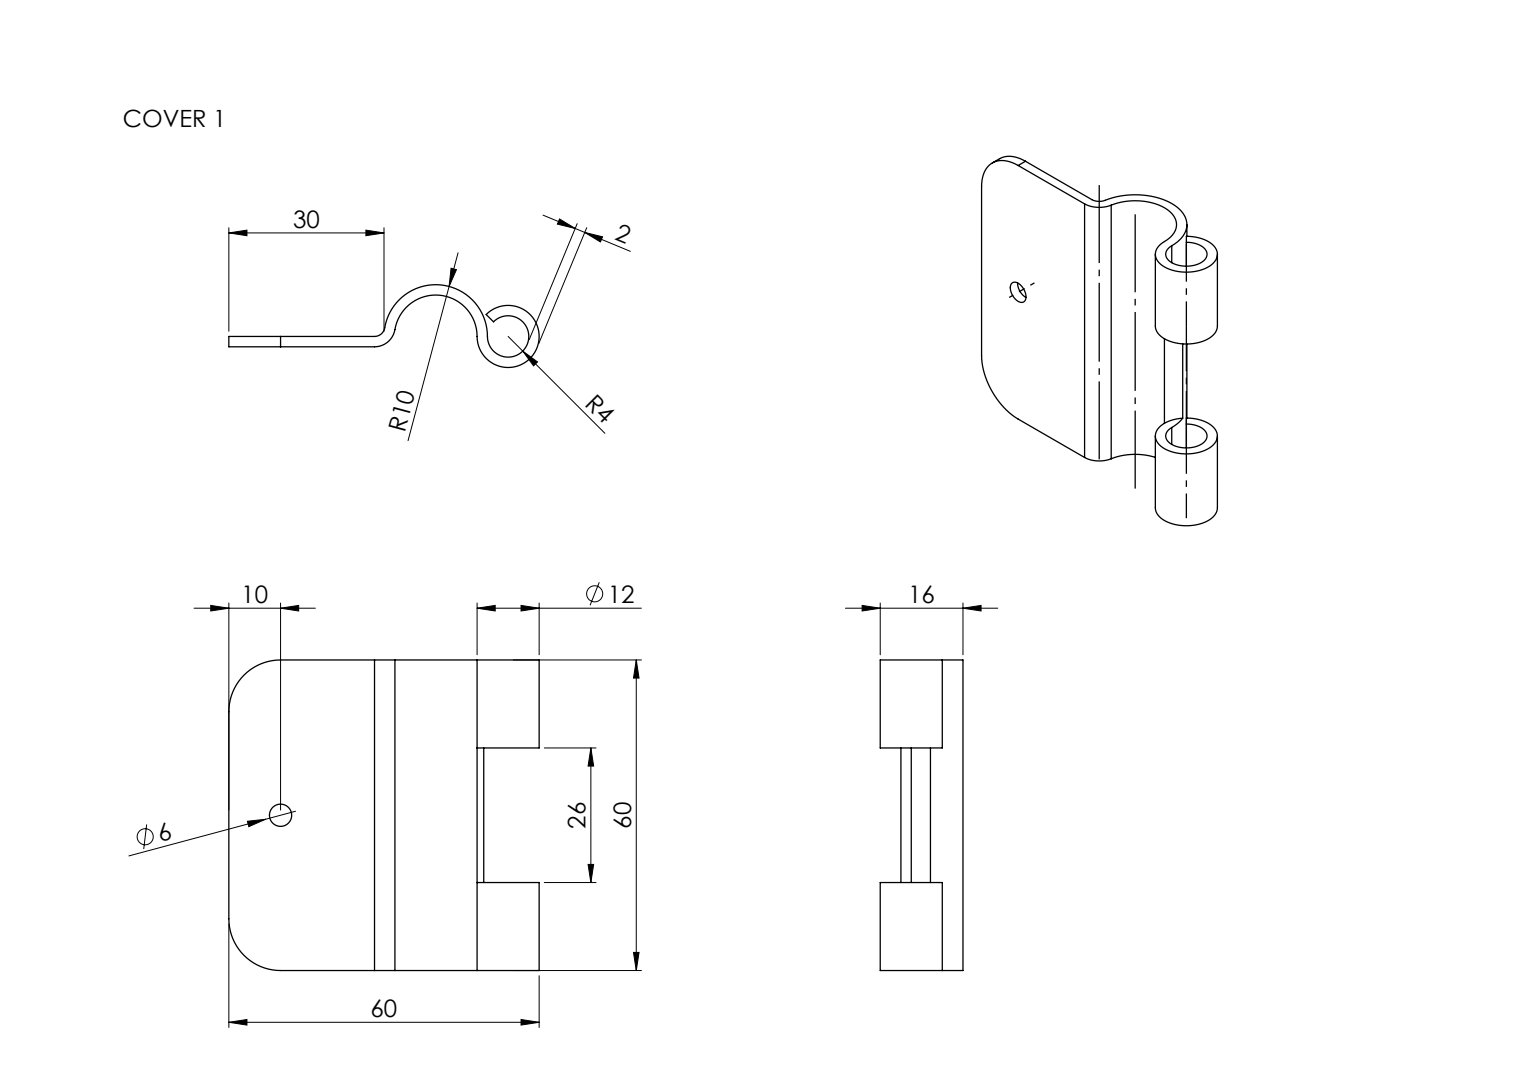
ISO-10303-21;
HEADER;
FILE_DESCRIPTION (('STEP AP214'),
    '1' );
FILE_NAME ('cover 1.step',
    '2026-10-03T20:08:58',
    ( '' ),
    ( '' ),
    'SwSTEP 2.0',
    'SolidWorks 2026',
    '' );
FILE_SCHEMA (( 'AUTOMOTIVE_DESIGN' ));
ENDSEC;

DATA;
#10=VECTOR ( 'NONE', #8821, 1000.000000000000000 ) ;
#24=LINE ( 'NONE', #10641, #9116 ) ;
#29=ORIENTED_EDGE ( 'NONE', *, *, #11225, .F. ) ;
#40=LINE ( 'NONE', #5122, #406 ) ;
#42=AXIS2_PLACEMENT_3D ( 'NONE', #12709, #3754, #3875 ) ;
#45=AXIS2_PLACEMENT_3D ( 'NONE', #142, #4066, #10040 ) ;
#48=DIRECTION ( 'NONE',  ( -0.000000000000000000, -1.000000000000000000, -0.000000000000000000 ) ) ;
#50=ORIENTED_EDGE ( 'NONE', *, *, #4393, .F. ) ;
#63=CARTESIAN_POINT ( 'NONE',  ( 14.00000000000000000, 12.99999999999999822, 0.000000000000000000 ) ) ;
#75=CARTESIAN_POINT ( 'NONE',  ( -11.83215956619923226, -30.00000000000000000, -4.336808689942017736E-16 ) ) ;
#77=DIRECTION ( 'NONE',  ( 0.000000000000000000, 0.000000000000000000, 1.000000000000000000 ) ) ;
#139=DIRECTION ( 'NONE',  ( 0.000000000000000000, 0.000000000000000000, -1.000000000000000000 ) ) ;
#142=CARTESIAN_POINT ( 'NONE',  ( 14.00000000000000000, 13.00000000000000000, 0.000000000000000000 ) ) ;
#148=CARTESIAN_POINT ( 'NONE',  ( 14.00000000000000000, -13.00000000000000000, 0.000000000000000000 ) ) ;
#158=ORIENTED_EDGE ( 'NONE', *, *, #7731, .T. ) ;
#171=AXIS2_PLACEMENT_3D ( 'NONE', #7633, #11626, #11439 ) ;
#181=ORIENTED_EDGE ( 'NONE', *, *, #9473, .F. ) ;
#187=AXIS2_PLACEMENT_3D ( 'NONE', #3419, #6498, #628 ) ;
#234=CIRCLE ( 'NONE', #8869, 6.000000000000000888 ) ;
#235=VERTEX_POINT ( 'NONE', #4529 ) ;
#237=EDGE_LOOP ( 'NONE', ( #1805, #3324, #10150, #7771, #10592, #866 ) ) ;
#273=CARTESIAN_POINT ( 'NONE',  ( 0.000000000000000000, 30.00000000000000000, 0.000000000000000000 ) ) ;
#288=AXIS2_PLACEMENT_3D ( 'NONE', #9402, #7554, #2747 ) ;
#294=DIRECTION ( 'NONE',  ( 0.000000000000000000, 0.000000000000000000, -1.000000000000000000 ) ) ;
#301=EDGE_LOOP ( 'NONE', ( #811, #8757, #4299, #181 ) ) ;
#303=VERTEX_POINT ( 'NONE', #7427 ) ;
#305=DIRECTION ( 'NONE',  ( -0.000000000000000000, -1.000000000000000000, -0.000000000000000000 ) ) ;
#333=EDGE_CURVE ( 'NONE', #5304, #561, #531, .T. ) ;
#344=DIRECTION ( 'NONE',  ( 0.000000000000000000, 0.000000000000000000, -1.000000000000000000 ) ) ;
#358=DIRECTION ( 'NONE',  ( 0.000000000000000000, 0.000000000000000000, 1.000000000000000000 ) ) ;
#377=ADVANCED_FACE ( 'NONE', ( #8824 ), #11672, .F. ) ;
#395=CARTESIAN_POINT ( 'NONE',  ( 14.00000000000000000, 12.99999999999999822, -4.000000000000000000 ) ) ;
#399=ORIENTED_EDGE ( 'NONE', *, *, #1607, .F. ) ;
#406=VECTOR ( 'NONE', #8142, 1000.000000000000000 ) ;
#412=VERTEX_POINT ( 'NONE', #4779 ) ;
#436=CARTESIAN_POINT ( 'NONE',  ( -11.83215956619923226, 30.00000000000000000, -4.336808689942017736E-16 ) ) ;
#444=VERTEX_POINT ( 'NONE', #9653 ) ;
#464=DIRECTION ( 'NONE',  ( 0.000000000000000000, 0.000000000000000000, -1.000000000000000000 ) ) ;
#469=DIRECTION ( 'NONE',  ( -1.000000000000000000, 0.000000000000000000, 1.301042606982605074E-16 ) ) ;
#475=ORIENTED_EDGE ( 'NONE', *, *, #9984, .T. ) ;
#476=CIRCLE ( 'NONE', #5414, 10.00000000000000178 ) ;
#531=LINE ( 'NONE', #9277, #10738 ) ;
#532=ADVANCED_FACE ( 'NONE', ( #11863 ), #11017, .F. ) ;
#535=DIRECTION ( 'NONE',  ( -0.000000000000000000, -1.000000000000000000, -0.000000000000000000 ) ) ;
#536=FACE_OUTER_BOUND ( 'NONE', #5367, .T. ) ;
#549=FACE_OUTER_BOUND ( 'NONE', #3644, .T. ) ;
#556=ORIENTED_EDGE ( 'NONE', *, *, #9689, .T. ) ;
#561=VERTEX_POINT ( 'NONE', #3052 ) ;
#617=ORIENTED_EDGE ( 'NONE', *, *, #7288, .T. ) ;
#628=DIRECTION ( 'NONE',  ( -1.000000000000000000, 0.000000000000000000, 1.159061634649218351E-16 ) ) ;
#638=DIRECTION ( 'NONE',  ( 0.000000000000000000, 1.000000000000000000, 0.000000000000000000 ) ) ;
#661=LINE ( 'NONE', #3823, #6580 ) ;
#672=DIRECTION ( 'NONE',  ( 0.000000000000000000, 0.000000000000000000, 1.000000000000000000 ) ) ;
#688=FACE_OUTER_BOUND ( 'NONE', #7012, .T. ) ;
#698=ORIENTED_EDGE ( 'NONE', *, *, #11571, .F. ) ;
#707=LINE ( 'NONE', #10430, #5346 ) ;
#711=VERTEX_POINT ( 'NONE', #7351 ) ;
#721=CARTESIAN_POINT ( 'NONE',  ( 14.00000000000000000, -12.99999999999999822, 0.000000000000000000 ) ) ;
#722=DIRECTION ( 'NONE',  ( -0.000000000000000000, 1.000000000000000000, 0.000000000000000000 ) ) ;
#727=CARTESIAN_POINT ( 'NONE',  ( 14.00000000000000000, -13.00000000000000000, 0.000000000000000000 ) ) ;
#729=VECTOR ( 'NONE', #11677, 1000.000000000000000 ) ;
#744=DIRECTION ( 'NONE',  ( 1.000000000000000000, 0.000000000000000000, 0.000000000000000000 ) ) ;
#751=AXIS2_PLACEMENT_3D ( 'NONE', #5443, #1637, #672 ) ;
#768=AXIS2_PLACEMENT_3D ( 'NONE', #5005, #48, #5840 ) ;
#771=DIRECTION ( 'NONE',  ( -0.000000000000000000, -1.000000000000000000, -0.000000000000000000 ) ) ;
#785=DIRECTION ( 'NONE',  ( 0.000000000000000000, 1.000000000000000000, 0.000000000000000000 ) ) ;
#803=VERTEX_POINT ( 'NONE', #3678 ) ;
#811=ORIENTED_EDGE ( 'NONE', *, *, #11377, .F. ) ;
#816=AXIS2_PLACEMENT_3D ( 'NONE', #12029, #3339, #7260 ) ;
#829=ORIENTED_EDGE ( 'NONE', *, *, #12238, .T. ) ;
#847=DIRECTION ( 'NONE',  ( 0.000000000000000000, 1.000000000000000000, 0.000000000000000000 ) ) ;
#866=ORIENTED_EDGE ( 'NONE', *, *, #11872, .F. ) ;
#898=AXIS2_PLACEMENT_3D ( 'NONE', #10933, #5615, #7679 ) ;
#924=DIRECTION ( 'NONE',  ( -0.000000000000000000, -1.000000000000000000, -0.000000000000000000 ) ) ;
#958=DIRECTION ( 'NONE',  ( 0.000000000000000000, 1.000000000000000000, 0.000000000000000000 ) ) ;
#971=LINE ( 'NONE', #75, #10203 ) ;
#974=LINE ( 'NONE', #5040, #7987 ) ;
#975=CIRCLE ( 'NONE', #6121, 2.000000000000000888 ) ;
#989=ORIENTED_EDGE ( 'NONE', *, *, #9398, .F. ) ;
#991=CARTESIAN_POINT ( 'NONE',  ( -30.00000000000000000, -19.99999999999999645, 0.000000000000000000 ) ) ;
#993=AXIS2_PLACEMENT_3D ( 'NONE', #148, #7994, #12663 ) ;
#998=DIRECTION ( 'NONE',  ( 0.000000000000000000, 0.000000000000000000, 1.000000000000000000 ) ) ;
#1000=ADVANCED_FACE ( 'NONE', ( #9168 ), #11180, .F. ) ;
#1016=ORIENTED_EDGE ( 'NONE', *, *, #5333, .F. ) ;
#1021=CIRCLE ( 'NONE', #8427, 4.000000000000000000 ) ;
#1034=CARTESIAN_POINT ( 'NONE',  ( -7.888106377466153063, -30.00000000000000000, -1.333333333333333703 ) ) ;
#1048=ADVANCED_FACE ( 'NONE', ( #9113 ), #5377, .T. ) ;
#1049=ADVANCED_FACE ( 'NONE', ( #8082 ), #8340, .T. ) ;
#1083=ADVANCED_FACE ( 'NONE', ( #549 ), #5630, .T. ) ;
#1111=ORIENTED_EDGE ( 'NONE', *, *, #9158, .T. ) ;
#1112=AXIS2_PLACEMENT_3D ( 'NONE', #1368, #344, #1244 ) ;
#1120=ORIENTED_EDGE ( 'NONE', *, *, #3514, .F. ) ;
#1127=ADVANCED_FACE ( 'NONE', ( #5693 ), #5574, .F. ) ;
#1155=ORIENTED_EDGE ( 'NONE', *, *, #3496, .F. ) ;
#1184=ORIENTED_EDGE ( 'NONE', *, *, #4506, .F. ) ;
#1193=FACE_BOUND ( 'NONE', #4343, .T. ) ;
#1200=ORIENTED_EDGE ( 'NONE', *, *, #2352, .F. ) ;
#1204=DIRECTION ( 'NONE',  ( -0.000000000000000000, -1.000000000000000000, -0.000000000000000000 ) ) ;
#1217=CARTESIAN_POINT ( 'NONE',  ( 9.999999999999998224, 30.00000000000000000, -6.123233995736765296E-16 ) ) ;
#1218=ORIENTED_EDGE ( 'NONE', *, *, #5875, .F. ) ;
#1242=CARTESIAN_POINT ( 'NONE',  ( -11.83215956619923226, -30.00000000000000000, -2.000000000000000888 ) ) ;
#1244=DIRECTION ( 'NONE',  ( -1.000000000000000000, 0.000000000000000000, 0.000000000000000000 ) ) ;
#1252=ORIENTED_EDGE ( 'NONE', *, *, #11293, .F. ) ;
#1255=PRESENTATION_STYLE_ASSIGNMENT (( #6281 ) ) ;
#1259=ADVANCED_FACE ( 'NONE', ( #4856 ), #6861, .F. ) ;
#1268=VECTOR ( 'NONE', #3945, 1000.000000000000000 ) ;
#1275=EDGE_CURVE ( 'NONE', #10532, #8740, #9012, .T. ) ;
#1283=DIRECTION ( 'NONE',  ( -0.000000000000000000, -1.000000000000000000, -0.000000000000000000 ) ) ;
#1287=ADVANCED_FACE ( 'NONE', ( #4920 ), #8781, .F. ) ;
#1288=CARTESIAN_POINT ( 'NONE',  ( 14.00000000000000000, -13.00000000000000000, 0.000000000000000000 ) ) ;
#1293=FACE_OUTER_BOUND ( 'NONE', #6936, .T. ) ;
#1307=APPLICATION_CONTEXT ( 'automotive_design' ) ;
#1309=CARTESIAN_POINT ( 'NONE',  ( -30.00000000000000000, 0.000000000000000000, 2.000000000000001776 ) ) ;
#1321=DIRECTION ( 'NONE',  ( 0.000000000000000000, 0.000000000000000000, -1.000000000000000000 ) ) ;
#1357=FACE_OUTER_BOUND ( 'NONE', #4922, .T. ) ;
#1368=CARTESIAN_POINT ( 'NONE',  ( -30.00000000000000000, 19.99999999999999645, 2.000000000000003109 ) ) ;
#1384=DIRECTION ( 'NONE',  ( -0.000000000000000000, -1.000000000000000000, -0.000000000000000000 ) ) ;
#1385=CARTESIAN_POINT ( 'NONE',  ( -27.85000000000000497, 2.632990618166801840E-16, 3.477184903947654954E-15 ) ) ;
#1404=CARTESIAN_POINT ( 'NONE',  ( -27.85000000000000853, 2.632990618166797895E-16, 2.185182530847200403E-15 ) ) ;
#1414=AXIS2_PLACEMENT_3D ( 'NONE', #436, #9498, #8356 ) ;
#1424=AXIS2_PLACEMENT_3D ( 'NONE', #12463, #7493, #4722 ) ;
#1426=AXIS2_PLACEMENT_3D ( 'NONE', #9293, #1384, #294 ) ;
#1444=CIRCLE ( 'NONE', #11915, 9.999999999999998224 ) ;
#1450=DIRECTION ( 'NONE',  ( -0.000000000000000000, -1.000000000000000000, -0.000000000000000000 ) ) ;
#1458=VERTEX_POINT ( 'NONE', #3664 ) ;
#1464=FACE_BOUND ( 'NONE', #5052, .T. ) ;
#1498=AXIS2_PLACEMENT_3D ( 'NONE', #11593, #2721, #9508 ) ;
#1523=ORIENTED_EDGE ( 'NONE', *, *, #4552, .F. ) ;
#1562=CYLINDRICAL_SURFACE ( 'NONE', #4873, 6.000000000000000000 ) ;
#1575=AXIS2_PLACEMENT_3D ( 'NONE', #1288, #10948, #10100 ) ;
#1580=CARTESIAN_POINT ( 'NONE',  ( 11.17157287525379772, 12.99999999999999822, -2.828427124746177856 ) ) ;
#1584=VERTEX_POINT ( 'NONE', #3083 ) ;
#1586=EDGE_LOOP ( 'NONE', ( #3626, #12343, #10983, #4232 ) ) ;
#1594=CARTESIAN_POINT ( 'NONE',  ( -40.00000000000000000, 19.99999999999999645, 2.000000000000003109 ) ) ;
#1607=EDGE_CURVE ( 'NONE', #3905, #2770, #8981, .T. ) ;
#1625=FACE_OUTER_BOUND ( 'NONE', #12477, .T. ) ;
#1637=DIRECTION ( 'NONE',  ( 0.000000000000000000, 1.000000000000000000, 0.000000000000000000 ) ) ;
#1641=EDGE_CURVE ( 'NONE', #3905, #1917, #6781, .T. ) ;
#1652=ORIENTED_EDGE ( 'NONE', *, *, #9989, .F. ) ;
#1655=SURFACE_SIDE_STYLE ('',( #4680 ) ) ;
#1661=VERTEX_POINT ( 'NONE', #4939 ) ;
#1670=CARTESIAN_POINT ( 'NONE',  ( 14.00000000000000000, -30.00000000000000000, 0.000000000000000000 ) ) ;
#1686=CIRCLE ( 'NONE', #45, 6.000000000000000888 ) ;
#1691=DIRECTION ( 'NONE',  ( -0.000000000000000000, -1.000000000000000000, -0.000000000000000000 ) ) ;
#1701=AXIS2_PLACEMENT_3D ( 'NONE', #5779, #5011, #9759 ) ;
#1790=AXIS2_PLACEMENT_3D ( 'NONE', #3328, #7245, #11163 ) ;
#1805=ORIENTED_EDGE ( 'NONE', *, *, #9881, .F. ) ;
#1817=DIRECTION ( 'NONE',  ( 0.000000000000000000, 0.000000000000000000, -1.000000000000000000 ) ) ;
#1820=EDGE_CURVE ( 'NONE', #6210, #11779, #1021, .T. ) ;
#1823=EDGE_LOOP ( 'NONE', ( #12079, #4616, #6876, #7646, #2549, #2027, #4556, #1218, #11515 ) ) ;
#1840=VECTOR ( 'NONE', #10679, 1000.000000000000000 ) ;
#1859=EDGE_CURVE ( 'NONE', #7604, #11454, #8226, .T. ) ;
#1885=AXIS2_PLACEMENT_3D ( 'NONE', #7237, #12196, #5357 ) ;
#1890=CARTESIAN_POINT ( 'NONE',  ( 14.00000000000000000, 30.00000000000000000, 0.000000000000000000 ) ) ;
#1895=CIRCLE ( 'NONE', #2324, 2.149999999999992362 ) ;
#1910=DIRECTION ( 'NONE',  ( 0.000000000000000000, -1.000000000000000000, 0.000000000000000000 ) ) ;
#1917=VERTEX_POINT ( 'NONE', #7123 ) ;
#1919=VECTOR ( 'NONE', #11565, 1000.000000000000000 ) ;
#1924=DIRECTION ( 'NONE',  ( -0.000000000000000000, -1.000000000000000000, -0.000000000000000000 ) ) ;
#1926=LINE ( 'NONE', #7854, #1840 ) ;
#1942=EDGE_CURVE ( 'NONE', #5074, #303, #40, .T. ) ;
#1953=CARTESIAN_POINT ( 'NONE',  ( -32.14999999999998437, 0.000000000000000000, 2.185182530847200403E-15 ) ) ;
#1960=AXIS2_PLACEMENT_3D ( 'NONE', #10965, #8263, #2155 ) ;
#1971=EDGE_LOOP ( 'NONE', ( #7157, #9270, #9490, #4872 ) ) ;
#1976=ORIENTED_EDGE ( 'NONE', *, *, #4473, .F. ) ;
#2027=ORIENTED_EDGE ( 'NONE', *, *, #11377, .T. ) ;
#2033=VECTOR ( 'NONE', #5157, 1000.000000000000000 ) ;
#2042=CIRCLE ( 'NONE', #6789, 6.000000000000000000 ) ;
#2057=CARTESIAN_POINT ( 'NONE',  ( 9.757359312880696578, 30.00000000000000000, -4.242640687119267007 ) ) ;
#2066=LINE ( 'NONE', #11735, #10 ) ;
#2073=LINE ( 'NONE', #5995, #4306 ) ;
#2106=PLANE ( 'NONE',  #5291 ) ;
#2117=CARTESIAN_POINT ( 'NONE',  ( -30.00000000000000000, 0.000000000000000000, 2.185182530847200403E-15 ) ) ;
#2155=DIRECTION ( 'NONE',  ( 0.000000000000000000, 0.000000000000000000, -1.000000000000000000 ) ) ;
#2157=LINE ( 'NONE', #3013, #9658 ) ;
#2158=ORIENTED_EDGE ( 'NONE', *, *, #3957, .T. ) ;
#2174=DIRECTION ( 'NONE',  ( -0.000000000000000000, -0.000000000000000000, -1.000000000000000000 ) ) ;
#2183=EDGE_LOOP ( 'NONE', ( #11415, #8143, #11917, #10065 ) ) ;
#2184=EDGE_CURVE ( 'NONE', #9120, #8530, #2066, .T. ) ;
#2214=ORIENTED_EDGE ( 'NONE', *, *, #6084, .F. ) ;
#2240=ORIENTED_EDGE ( 'NONE', *, *, #1641, .F. ) ;
#2258=DIRECTION ( 'NONE',  ( 1.000000000000000000, 0.000000000000000000, 0.000000000000000000 ) ) ;
#2265=PLANE ( 'NONE',  #4114 ) ;
#2284=COLOUR_RGB ( '', 0.72549020, 0.75294118, 0.79215686) ;
#2299=ORIENTED_EDGE ( 'NONE', *, *, #5405, .F. ) ;
#2310=ORIENTED_EDGE ( 'NONE', *, *, #5875, .T. ) ;
#2324=AXIS2_PLACEMENT_3D ( 'NONE', #9320, #4378, #10287 ) ;
#2332=AXIS2_PLACEMENT_3D ( 'NONE', #1670, #638, #4577 ) ;
#2333=CARTESIAN_POINT ( 'NONE',  ( 14.00000000000000000, 30.00000000000000000, 0.000000000000000000 ) ) ;
#2336=FACE_OUTER_BOUND ( 'NONE', #3673, .T. ) ;
#2352=EDGE_CURVE ( 'NONE', #1661, #235, #12058, .T. ) ;
#2381=ORIENTED_EDGE ( 'NONE', *, *, #2850, .T. ) ;
#2382=DIRECTION ( 'NONE',  ( 0.000000000000000000, 0.000000000000000000, 1.000000000000000000 ) ) ;
#2387=ADVANCED_FACE ( 'NONE', ( #4252 ), #2265, .F. ) ;
#2391=ORIENTED_EDGE ( 'NONE', *, *, #2184, .T. ) ;
#2392=AXIS2_PLACEMENT_3D ( 'NONE', #6722, #12712, #5872 ) ;
#2416=PRODUCT_DEFINITION_FORMATION_WITH_SPECIFIED_SOURCE ( 'ANY', '', #6601, .NOT_KNOWN. ) ;
#2417=AXIS2_PLACEMENT_3D ( 'NONE', #721, #847, #10566 ) ;
#2426=VECTOR ( 'NONE', #3154, 1000.000000000000000 ) ;
#2438=ORIENTED_EDGE ( 'NONE', *, *, #10969, .T. ) ;
#2444=FACE_OUTER_BOUND ( 'NONE', #7944, .T. ) ;
#2461=AXIS2_PLACEMENT_3D ( 'NONE', #8419, #9369, #7579 ) ;
#2465=FACE_OUTER_BOUND ( 'NONE', #10736, .T. ) ;
#2476=CARTESIAN_POINT ( 'NONE',  ( 14.00000000000000000, 30.00000000000000000, 6.000000000000000000 ) ) ;
#2493=CARTESIAN_POINT ( 'NONE',  ( -30.00000000000000000, -19.99999999999999645, 2.000000000000001776 ) ) ;
#2495=DIRECTION ( 'NONE',  ( 0.000000000000000000, 0.000000000000000000, -1.000000000000000000 ) ) ;
#2509=DIRECTION ( 'NONE',  ( 0.000000000000000000, 0.000000000000000000, -1.000000000000000000 ) ) ;
#2537=CIRCLE ( 'NONE', #2332, 6.000000000000000000 ) ;
#2549=ORIENTED_EDGE ( 'NONE', *, *, #5470, .T. ) ;
#2572=ORIENTED_EDGE ( 'NONE', *, *, #7361, .F. ) ;
#2574=CARTESIAN_POINT ( 'NONE',  ( 0.000000000000000000, -30.00000000000000000, 0.000000000000000000 ) ) ;
#2600=ORIENTED_EDGE ( 'NONE', *, *, #7623, .F. ) ;
#2611=STYLED_ITEM ( 'NONE', ( #1255 ), #5784 ) ;
#2664=DIRECTION ( 'NONE',  ( -0.000000000000000000, -1.000000000000000000, -0.000000000000000000 ) ) ;
#2676=CARTESIAN_POINT ( 'NONE',  ( 11.17157287525379772, 30.00000000000000000, -2.828427124746177856 ) ) ;
#2704=ORIENTED_EDGE ( 'NONE', *, *, #3659, .F. ) ;
#2716=CARTESIAN_POINT ( 'NONE',  ( 14.00000000000000000, -30.00000000000000000, 6.000000000000000000 ) ) ;
#2721=DIRECTION ( 'NONE',  ( 0.000000000000000000, 1.000000000000000000, 0.000000000000000000 ) ) ;
#2745=DIRECTION ( 'NONE',  ( 1.000000000000000000, 0.000000000000000000, 0.000000000000000000 ) ) ;
#2747=DIRECTION ( 'NONE',  ( -1.000000000000000000, 0.000000000000000000, 0.000000000000000000 ) ) ;
#2751=EDGE_CURVE ( 'NONE', #11755, #9393, #12335, .T. ) ;
#2770=VERTEX_POINT ( 'NONE', #4043 ) ;
#2782=VERTEX_POINT ( 'NONE', #5267 ) ;
#2805=DIRECTION ( 'NONE',  ( 1.000000000000000000, 0.000000000000000000, -1.159061634649218351E-16 ) ) ;
#2809=DIRECTION ( 'NONE',  ( -0.7071067811865504593, 0.000000000000000000, -0.7071067811865445751 ) ) ;
#2810=ADVANCED_FACE ( 'NONE', ( #8032 ), #11066, .T. ) ;
#2818=VERTEX_POINT ( 'NONE', #9125 ) ;
#2843=ADVANCED_FACE ( 'NONE', ( #1464, #2444 ), #5588, .T. ) ;
#2850=EDGE_CURVE ( 'NONE', #5717, #8530, #1444, .T. ) ;
#2878=ADVANCED_FACE ( 'NONE', ( #688 ), #11522, .F. ) ;
#2901=CARTESIAN_POINT ( 'NONE',  ( 14.00000000000000000, -13.00000000000000000, 0.000000000000000000 ) ) ;
#2904=PRODUCT_DEFINITION ( 'UNKNOWN', '', #2416, #10936 ) ;
#2917=VECTOR ( 'NONE', #9738, 1000.000000000000000 ) ;
#2921=EDGE_CURVE ( 'NONE', #561, #2818, #5738, .T. ) ;
#2937=CARTESIAN_POINT ( 'NONE',  ( 14.00000000000000000, 30.00000000000000000, 4.000000000000000000 ) ) ;
#2941=VERTEX_POINT ( 'NONE', #5525 ) ;
#2943=DIRECTION ( 'NONE',  ( -0.000000000000000000, -1.000000000000000000, -0.000000000000000000 ) ) ;
#2953=ORIENTED_EDGE ( 'NONE', *, *, #9013, .F. ) ;
#2970=ORIENTED_EDGE ( 'NONE', *, *, #1859, .T. ) ;
#2976=ORIENTED_EDGE ( 'NONE', *, *, #4473, .T. ) ;
#2980=DIRECTION ( 'NONE',  ( 0.000000000000000000, 0.000000000000000000, 1.000000000000000000 ) ) ;
#3013=CARTESIAN_POINT ( 'NONE',  ( -7.888106377466153063, 30.00000000000000000, -1.333333333333333703 ) ) ;
#3023=VERTEX_POINT ( 'NONE', #12618 ) ;
#3032=ORIENTED_EDGE ( 'NONE', *, *, #5231, .T. ) ;
#3042=AXIS2_PLACEMENT_3D ( 'NONE', #3819, #3939, #6595 ) ;
#3052=CARTESIAN_POINT ( 'NONE',  ( -29.99999999999999289, -30.00000000000000000, 1.672083814130525448E-15 ) ) ;
#3054=EDGE_CURVE ( 'NONE', #803, #11695, #6235, .T. ) ;
#3070=EDGE_CURVE ( 'NONE', #3108, #11779, #5837, .T. ) ;
#3071=CARTESIAN_POINT ( 'NONE',  ( 0.000000000000000000, -30.00000000000000000, -9.999999999999998224 ) ) ;
#3082=VERTEX_POINT ( 'NONE', #10788 ) ;
#3083=CARTESIAN_POINT ( 'NONE',  ( 9.999999999999998224, -30.00000000000000000, -6.123233995736765296E-16 ) ) ;
#3085=ORIENTED_EDGE ( 'NONE', *, *, #6575, .T. ) ;
#3092=ORIENTED_EDGE ( 'NONE', *, *, #4506, .T. ) ;
#3103=CIRCLE ( 'NONE', #11936, 6.000000000000000000 ) ;
#3108=VERTEX_POINT ( 'NONE', #7649 ) ;
#3125=VECTOR ( 'NONE', #11827, 1000.000000000000000 ) ;
#3138=VECTOR ( 'NONE', #2664, 1000.000000000000000 ) ;
#3154=DIRECTION ( 'NONE',  ( -0.000000000000000000, -1.000000000000000000, -0.000000000000000000 ) ) ;
#3174=DIRECTION ( 'NONE',  ( 0.000000000000000000, 1.000000000000000000, 0.000000000000000000 ) ) ;
#3177=CIRCLE ( 'NONE', #5625, 7.999999999999998224 ) ;
#3197=DIRECTION ( 'NONE',  ( 0.000000000000000000, 1.000000000000000000, 0.000000000000000000 ) ) ;
#3245=DIRECTION ( 'NONE',  ( -1.000000000000000000, 0.000000000000000000, 0.000000000000000000 ) ) ;
#3247=CIRCLE ( 'NONE', #3042, 6.000000000000000000 ) ;
#3255=VECTOR ( 'NONE', #5993, 1000.000000000000000 ) ;
#3262=DIRECTION ( 'NONE',  ( 1.000000000000000000, 0.000000000000000000, 0.000000000000000000 ) ) ;
#3265=CIRCLE ( 'NONE', #10433, 9.999999999999998224 ) ;
#3284=ORIENTED_EDGE ( 'NONE', *, *, #12203, .T. ) ;
#3296=CARTESIAN_POINT ( 'NONE',  ( 11.17157287525379772, -12.99999999999999822, -2.828427124746177856 ) ) ;
#3302=CARTESIAN_POINT ( 'NONE',  ( -40.00000000000000000, 19.99999999999999645, 2.831145448779744488E-15 ) ) ;
#3318=DIRECTION ( 'NONE',  ( 0.000000000000000000, 1.000000000000000000, 0.000000000000000000 ) ) ;
#3320=CARTESIAN_POINT ( 'NONE',  ( -11.83215956619923226, 30.00000000000000000, 2.000000000000000000 ) ) ;
#3324=ORIENTED_EDGE ( 'NONE', *, *, #7361, .T. ) ;
#3328=CARTESIAN_POINT ( 'NONE',  ( 0.000000000000000000, 30.00000000000000000, 0.000000000000000000 ) ) ;
#3339=DIRECTION ( 'NONE',  ( -0.000000000000000000, -1.000000000000000000, -0.000000000000000000 ) ) ;
#3340=DIRECTION ( 'NONE',  ( -1.159061634649218351E-16, 0.000000000000000000, -1.000000000000000000 ) ) ;
#3376=CARTESIAN_POINT ( 'NONE',  ( 0.000000000000000000, 30.00000000000000000, -9.999999999999998224 ) ) ;
#3377=ORIENTED_EDGE ( 'NONE', *, *, #11293, .T. ) ;
#3381=EDGE_CURVE ( 'NONE', #235, #5304, #476, .T. ) ;
#3419=CARTESIAN_POINT ( 'NONE',  ( -30.00000000000000000, -19.99999999999999645, 1.672083814130526039E-15 ) ) ;
#3435=LINE ( 'NONE', #7353, #4862 ) ;
#3440=DIRECTION ( 'NONE',  ( -0.000000000000000000, -1.000000000000000000, -0.000000000000000000 ) ) ;
#3449=FACE_OUTER_BOUND ( 'NONE', #301, .T. ) ;
#3464=ADVANCED_FACE ( 'NONE', ( #3829 ), #6609, .F. ) ;
#3488=DIRECTION ( 'NONE',  ( -1.000000000000000000, 0.000000000000000000, 0.000000000000000000 ) ) ;
#3496=EDGE_CURVE ( 'NONE', #12099, #5977, #24, .T. ) ;
#3504=ORIENTED_EDGE ( 'NONE', *, *, #8796, .F. ) ;
#3508=CARTESIAN_POINT ( 'NONE',  ( 14.00000000000000000, 30.00000000000000000, 0.000000000000000000 ) ) ;
#3514=EDGE_CURVE ( 'NONE', #5304, #8798, #7631, .T. ) ;
#3530=EDGE_LOOP ( 'NONE', ( #3597, #9990, #8842, #11421 ) ) ;
#3537=ORIENTED_EDGE ( 'NONE', *, *, #4198, .F. ) ;
#3567=ORIENTED_EDGE ( 'NONE', *, *, #7143, .T. ) ;
#3574=VECTOR ( 'NONE', #12296, 1000.000000000000000 ) ;
#3582=ORIENTED_EDGE ( 'NONE', *, *, #10353, .T. ) ;
#3593=ORIENTED_EDGE ( 'NONE', *, *, #7143, .F. ) ;
#3597=ORIENTED_EDGE ( 'NONE', *, *, #12203, .F. ) ;
#3626=ORIENTED_EDGE ( 'NONE', *, *, #5180, .F. ) ;
#3638=UNCERTAINTY_MEASURE_WITH_UNIT (LENGTH_MEASURE( 1.000000000000000082E-05 ), #10533, 'distance_accuracy_value', 'NONE');
#3644=EDGE_LOOP ( 'NONE', ( #10651, #8593, #5758, #8809 ) ) ;
#3659=EDGE_CURVE ( 'NONE', #1458, #2782, #3177, .T. ) ;
#3664=CARTESIAN_POINT ( 'NONE',  ( -7.888106377466153063, 30.00000000000000000, -1.333333333333333703 ) ) ;
#3673=EDGE_LOOP ( 'NONE', ( #4612, #9882, #9043, #10462 ) ) ;
#3678=CARTESIAN_POINT ( 'NONE',  ( 14.00000000000000000, 12.99999999999999822, 4.000000000000000000 ) ) ;
#3702=DIRECTION ( 'NONE',  ( 0.000000000000000000, 1.000000000000000000, 0.000000000000000000 ) ) ;
#3711=VECTOR ( 'NONE', #6854, 1000.000000000000000 ) ;
#3754=DIRECTION ( 'NONE',  ( -0.000000000000000000, -1.000000000000000000, -0.000000000000000000 ) ) ;
#3758=CARTESIAN_POINT ( 'NONE',  ( 0.000000000000000000, -30.00000000000000000, 0.000000000000000000 ) ) ;
#3776=ORIENTED_EDGE ( 'NONE', *, *, #5299, .F. ) ;
#3789=CARTESIAN_POINT ( 'NONE',  ( 0.000000000000000000, 30.00000000000000000, 0.000000000000000000 ) ) ;
#3819=CARTESIAN_POINT ( 'NONE',  ( 14.00000000000000000, 30.00000000000000000, 0.000000000000000000 ) ) ;
#3823=CARTESIAN_POINT ( 'NONE',  ( 11.17157287525379772, 30.00000000000000000, -2.828427124746177856 ) ) ;
#3829=FACE_OUTER_BOUND ( 'NONE', #11908, .T. ) ;
#3839=ORIENTED_EDGE ( 'NONE', *, *, #7448, .F. ) ;
#3846=ORIENTED_EDGE ( 'NONE', *, *, #1942, .F. ) ;
#3861=VERTEX_POINT ( 'NONE', #8578 ) ;
#3875=DIRECTION ( 'NONE',  ( 0.000000000000000000, 0.000000000000000000, -1.000000000000000000 ) ) ;
#3879=DIRECTION ( 'NONE',  ( 1.000000000000000000, 0.000000000000000000, 0.000000000000000000 ) ) ;
#3897=AXIS2_PLACEMENT_3D ( 'NONE', #11809, #5102, #139 ) ;
#3905=VERTEX_POINT ( 'NONE', #12585 ) ;
#3909=CIRCLE ( 'NONE', #6799, 4.000000000000000000 ) ;
#3923=VERTEX_POINT ( 'NONE', #4045 ) ;
#3939=DIRECTION ( 'NONE',  ( 0.000000000000000000, 1.000000000000000000, 0.000000000000000000 ) ) ;
#3945=DIRECTION ( 'NONE',  ( -0.000000000000000000, -0.000000000000000000, 1.000000000000000000 ) ) ;
#3957=EDGE_CURVE ( 'NONE', #11695, #711, #8923, .T. ) ;
#3968=CARTESIAN_POINT ( 'NONE',  ( 0.000000000000000000, -30.00000000000000000, 0.000000000000000000 ) ) ;
#3987=CYLINDRICAL_SURFACE ( 'NONE', #10792, 4.000000000000000000 ) ;
#4020=VERTEX_POINT ( 'NONE', #3296 ) ;
#4021=AXIS2_PLACEMENT_3D ( 'NONE', #1242, #4271, #12142 ) ;
#4043=CARTESIAN_POINT ( 'NONE',  ( 8.000000000000000000, -30.00000000000000000, -7.347880794884119736E-16 ) ) ;
#4045=CARTESIAN_POINT ( 'NONE',  ( 9.999999999999998224, 30.00000000000000000, -6.123233995736765296E-16 ) ) ;
#4066=DIRECTION ( 'NONE',  ( 0.000000000000000000, 1.000000000000000000, 0.000000000000000000 ) ) ;
#4094=LINE ( 'NONE', #12030, #2426 ) ;
#4114=AXIS2_PLACEMENT_3D ( 'NONE', #10944, #7286, #11212 ) ;
#4143=EDGE_LOOP ( 'NONE', ( #1120, #9739, #12659, #12338, #2381, #6160, #6958, #10639, #3567, #12272, #8998, #8819, #9422, #4803, #7145, #7439 ) ) ;
#4164=DIRECTION ( 'NONE',  ( 0.000000000000000000, 1.000000000000000000, 0.000000000000000000 ) ) ;
#4185=CARTESIAN_POINT ( 'NONE',  ( 14.00000000000000000, 13.00000000000000000, 0.000000000000000000 ) ) ;
#4198=EDGE_CURVE ( 'NONE', #1661, #9551, #10408, .T. ) ;
#4208=ORIENTED_EDGE ( 'NONE', *, *, #3054, .F. ) ;
#4216=AXIS2_PLACEMENT_3D ( 'NONE', #63, #958, #2980 ) ;
#4228=CIRCLE ( 'NONE', #4021, 4.000000000000000000 ) ;
#4232=ORIENTED_EDGE ( 'NONE', *, *, #8987, .F. ) ;
#4235=CARTESIAN_POINT ( 'NONE',  ( 11.17157287525379772, -30.00000000000000000, -2.828427124746177856 ) ) ;
#4237=EDGE_LOOP ( 'NONE', ( #3504, #10227, #11106, #1111, #4887, #11159, #5172, #4346, #12022, #1652, #5776, #7252, #6142, #50, #7426, #10177 ) ) ;
#4246=CARTESIAN_POINT ( 'NONE',  ( 14.00000000000000000, -30.00000000000000000, 0.000000000000000000 ) ) ;
#4249=DIRECTION ( 'NONE',  ( 0.000000000000000000, 1.000000000000000000, 0.000000000000000000 ) ) ;
#4252=FACE_OUTER_BOUND ( 'NONE', #4143, .T. ) ;
#4271=DIRECTION ( 'NONE',  ( 0.000000000000000000, 1.000000000000000000, 0.000000000000000000 ) ) ;
#4276=VERTEX_POINT ( 'NONE', #10540 ) ;
#4295=LINE ( 'NONE', #9306, #5212 ) ;
#4299=ORIENTED_EDGE ( 'NONE', *, *, #12320, .T. ) ;
#4306=VECTOR ( 'NONE', #7806, 1000.000000000000000 ) ;
#4328=EDGE_CURVE ( 'NONE', #11755, #7484, #11060, .T. ) ;
#4343=EDGE_LOOP ( 'NONE', ( #3377, #3284 ) ) ;
#4346=ORIENTED_EDGE ( 'NONE', *, *, #5180, .T. ) ;
#4359=ORIENTED_EDGE ( 'NONE', *, *, #9569, .T. ) ;
#4364=CARTESIAN_POINT ( 'NONE',  ( -9.860132971832690885, -30.00000000000000000, -1.666666666666667629 ) ) ;
#4366=APPLICATION_CONTEXT ( 'automotive_design' ) ;
#4370=DIRECTION ( 'NONE',  ( 0.000000000000000000, 1.000000000000000000, 0.000000000000000000 ) ) ;
#4377=ORIENTED_EDGE ( 'NONE', *, *, #9013, .T. ) ;
#4378=DIRECTION ( 'NONE',  ( -1.159061634649218351E-16, 0.000000000000000000, -1.000000000000000000 ) ) ;
#4393=EDGE_CURVE ( 'NONE', #9120, #3923, #3265, .T. ) ;
#4400=DIRECTION ( 'NONE',  ( 0.000000000000000000, 0.000000000000000000, -1.000000000000000000 ) ) ;
#4426=LINE ( 'NONE', #8351, #3574 ) ;
#4463=CARTESIAN_POINT ( 'NONE',  ( 14.00000000000000000, -30.00000000000000000, 4.000000000000000000 ) ) ;
#4473=EDGE_CURVE ( 'NONE', #9408, #412, #12100, .T. ) ;
#4478=ORIENTED_EDGE ( 'NONE', *, *, #7288, .F. ) ;
#4483=EDGE_CURVE ( 'NONE', #9770, #5717, #975, .T. ) ;
#4488=CARTESIAN_POINT ( 'NONE',  ( -40.00000000000000000, 30.00000000000000000, 2.831145448779744488E-15 ) ) ;
#4489=VERTEX_POINT ( 'NONE', #8022 ) ;
#4506=EDGE_CURVE ( 'NONE', #2782, #11454, #4094, .T. ) ;
#4513=AXIS2_PLACEMENT_3D ( 'NONE', #10931, #1204, #11980 ) ;
#4526=ADVANCED_FACE ( 'NONE', ( #1193, #6154 ), #2106, .F. ) ;
#4529=CARTESIAN_POINT ( 'NONE',  ( -40.00000000000000000, -19.99999999999999645, 2.000000000000003109 ) ) ;
#4531=CARTESIAN_POINT ( 'NONE',  ( 14.00000000000000000, 30.00000000000000000, 4.000000000000000000 ) ) ;
#4549=DIRECTION ( 'NONE',  ( -0.000000000000000000, -1.000000000000000000, -0.000000000000000000 ) ) ;
#4552=EDGE_CURVE ( 'NONE', #4276, #8365, #10987, .T. ) ;
#4556=ORIENTED_EDGE ( 'NONE', *, *, #9984, .F. ) ;
#4574=ORIENTED_EDGE ( 'NONE', *, *, #11571, .T. ) ;
#4576=EDGE_LOOP ( 'NONE', ( #1184, #2704, #11370, #2970 ) ) ;
#4577=DIRECTION ( 'NONE',  ( 1.000000000000000000, 0.000000000000000000, 0.000000000000000000 ) ) ;
#4612=ORIENTED_EDGE ( 'NONE', *, *, #7383, .T. ) ;
#4616=ORIENTED_EDGE ( 'NONE', *, *, #12238, .F. ) ;
#4629=CIRCLE ( 'NONE', #10779, 4.000000000000000000 ) ;
#4641=AXIS2_PLACEMENT_3D ( 'NONE', #11442, #12353, #4741 ) ;
#4644=PRODUCT_DEFINITION_SHAPE ( 'NONE', 'NONE',  #2904 ) ;
#4680=SURFACE_STYLE_FILL_AREA ( #10335 ) ;
#4714=AXIS2_PLACEMENT_3D ( 'NONE', #7018, #5329, #2382 ) ;
#4722=DIRECTION ( 'NONE',  ( 0.000000000000000000, 0.000000000000000000, 1.000000000000000000 ) ) ;
#4741=DIRECTION ( 'NONE',  ( 0.000000000000000000, 0.000000000000000000, 1.000000000000000000 ) ) ;
#4747=MECHANICAL_DESIGN_GEOMETRIC_PRESENTATION_REPRESENTATION('',(#11741),#5160);
#4751=SURFACE_STYLE_USAGE ( .BOTH. , #1655 ) ;
#4765=CIRCLE ( 'NONE', #5370, 2.149999999999992362 ) ;
#4779=CARTESIAN_POINT ( 'NONE',  ( 9.757359312880696578, 13.00000000000000000, -4.242640687119267895 ) ) ;
#4786=CIRCLE ( 'NONE', #6022, 2.149999999999985256 ) ;
#4803=ORIENTED_EDGE ( 'NONE', *, *, #7731, .F. ) ;
#4828=AXIS2_PLACEMENT_3D ( 'NONE', #7278, #4370, #11200 ) ;
#4835=VERTEX_POINT ( 'NONE', #1953 ) ;
#4844=AXIS2_PLACEMENT_3D ( 'NONE', #9985, #6139, #469 ) ;
#4856=FACE_OUTER_BOUND ( 'NONE', #11883, .T. ) ;
#4862=VECTOR ( 'NONE', #7231, 1000.000000000000000 ) ;
#4863=LINE ( 'NONE', #12730, #7831 ) ;
#4872=ORIENTED_EDGE ( 'NONE', *, *, #3957, .F. ) ;
#4873=AXIS2_PLACEMENT_3D ( 'NONE', #3508, #535, #4400 ) ;
#4887=ORIENTED_EDGE ( 'NONE', *, *, #3659, .T. ) ;
#4915=CARTESIAN_POINT ( 'NONE',  ( 14.00000000000000000, 30.00000000000000000, 0.000000000000000000 ) ) ;
#4920=FACE_OUTER_BOUND ( 'NONE', #10327, .T. ) ;
#4922=EDGE_LOOP ( 'NONE', ( #6338, #11445, #2976, #10317 ) ) ;
#4931=LINE ( 'NONE', #8851, #3125 ) ;
#4939=CARTESIAN_POINT ( 'NONE',  ( -40.00000000000000000, 19.99999999999999645, 2.000000000000003109 ) ) ;
#4960=ORIENTED_EDGE ( 'NONE', *, *, #10619, .T. ) ;
#4987=CARTESIAN_POINT ( 'NONE',  ( 8.000000000000000000, 30.00000000000000000, -7.347880794884119736E-16 ) ) ;
#5005=CARTESIAN_POINT ( 'NONE',  ( 0.000000000000000000, 12.99999999999999822, 0.000000000000000000 ) ) ;
#5011=DIRECTION ( 'NONE',  ( -0.000000000000000000, -0.000000000000000000, -1.000000000000000000 ) ) ;
#5020=EDGE_CURVE ( 'NONE', #2782, #6170, #11463, .T. ) ;
#5040=CARTESIAN_POINT ( 'NONE',  ( -11.83215956619923226, 30.00000000000000000, -4.336808689942017736E-16 ) ) ;
#5052=EDGE_LOOP ( 'NONE', ( #12492, #6427 ) ) ;
#5053=ADVANCED_FACE ( 'NONE', ( #3449 ), #1562, .T. ) ;
#5056=DIRECTION ( 'NONE',  ( -0.000000000000000000, -1.000000000000000000, -0.000000000000000000 ) ) ;
#5074=VERTEX_POINT ( 'NONE', #2476 ) ;
#5102=DIRECTION ( 'NONE',  ( 0.000000000000000000, -1.000000000000000000, 0.000000000000000000 ) ) ;
#5106=ORIENTED_EDGE ( 'NONE', *, *, #7627, .T. ) ;
#5109=AXIS2_PLACEMENT_3D ( 'NONE', #10187, #1450, #2495 ) ;
#5122=CARTESIAN_POINT ( 'NONE',  ( 14.00000000000000000, 30.00000000000000000, 6.000000000000000000 ) ) ;
#5130=( NAMED_UNIT ( * ) SI_UNIT ( $, .STERADIAN. ) SOLID_ANGLE_UNIT ( ) );
#5157=DIRECTION ( 'NONE',  ( -0.000000000000000000, -1.000000000000000000, -0.000000000000000000 ) ) ;
#5158=ORIENTED_EDGE ( 'NONE', *, *, #10844, .T. ) ;
#5159=CARTESIAN_POINT ( 'NONE',  ( -30.00000000000000000, 0.000000000000000000, 3.477184903947654954E-15 ) ) ;
#5160=( GEOMETRIC_REPRESENTATION_CONTEXT ( 3 ) GLOBAL_UNCERTAINTY_ASSIGNED_CONTEXT ( ( #11617 ) ) GLOBAL_UNIT_ASSIGNED_CONTEXT ( ( #12424, #11452, #12364 ) ) REPRESENTATION_CONTEXT ( 'NONE', 'WORKASPACE' ) );
#5172=ORIENTED_EDGE ( 'NONE', *, *, #6084, .T. ) ;
#5174=DIRECTION ( 'NONE',  ( 1.000000000000000000, 0.000000000000000000, 0.000000000000000000 ) ) ;
#5180=EDGE_CURVE ( 'NONE', #5074, #6567, #3247, .T. ) ;
#5188=ORIENTED_EDGE ( 'NONE', *, *, #2751, .T. ) ;
#5199=ORIENTED_EDGE ( 'NONE', *, *, #11225, .T. ) ;
#5212=VECTOR ( 'NONE', #305, 1000.000000000000000 ) ;
#5231=EDGE_CURVE ( 'NONE', #4489, #12605, #11669, .T. ) ;
#5255=DIRECTION ( 'NONE',  ( -0.000000000000000000, -1.000000000000000000, -0.000000000000000000 ) ) ;
#5267=CARTESIAN_POINT ( 'NONE',  ( 0.000000000000000000, 30.00000000000000000, -7.999999999999998224 ) ) ;
#5283=EDGE_CURVE ( 'NONE', #8740, #711, #6849, .T. ) ;
#5291=AXIS2_PLACEMENT_3D ( 'NONE', #7957, #3340, #10189 ) ;
#5299=EDGE_CURVE ( 'NONE', #9551, #12099, #10625, .T. ) ;
#5304=VERTEX_POINT ( 'NONE', #7922 ) ;
#5312=( LENGTH_UNIT ( ) NAMED_UNIT ( * ) SI_UNIT ( .MILLI., .METRE. ) );
#5329=DIRECTION ( 'NONE',  ( 0.000000000000000000, 1.000000000000000000, 0.000000000000000000 ) ) ;
#5333=EDGE_CURVE ( 'NONE', #2941, #3905, #12075, .T. ) ;
#5343=DIRECTION ( 'NONE',  ( -0.000000000000000000, -1.000000000000000000, -0.000000000000000000 ) ) ;
#5346=VECTOR ( 'NONE', #771, 1000.000000000000000 ) ;
#5357=DIRECTION ( 'NONE',  ( 0.000000000000000000, 0.000000000000000000, -1.000000000000000000 ) ) ;
#5367=EDGE_LOOP ( 'NONE', ( #11973, #4960, #3085, #989 ) ) ;
#5370=AXIS2_PLACEMENT_3D ( 'NONE', #1309, #5434, #9286 ) ;
#5377=CYLINDRICAL_SURFACE ( 'NONE', #1426, 9.999999999999998224 ) ;
#5405=EDGE_CURVE ( 'NONE', #6222, #803, #7033, .T. ) ;
#5414=AXIS2_PLACEMENT_3D ( 'NONE', #2493, #5442, #7320 ) ;
#5415=PLANE ( 'NONE',  #10469 ) ;
#5434=DIRECTION ( 'NONE',  ( -1.159061634649218351E-16, 0.000000000000000000, -1.000000000000000000 ) ) ;
#5437=CIRCLE ( 'NONE', #12650, 7.999999999999998224 ) ;
#5438=EDGE_LOOP ( 'NONE', ( #3032, #7643, #7528, #8879 ) ) ;
#5439=CIRCLE ( 'NONE', #4828, 6.000000000000000000 ) ;
#5442=DIRECTION ( 'NONE',  ( 1.159061634649218351E-16, -0.000000000000000000, 1.000000000000000000 ) ) ;
#5443=CARTESIAN_POINT ( 'NONE',  ( 14.00000000000000000, -12.99999999999999822, 0.000000000000000000 ) ) ;
#5470=EDGE_CURVE ( 'NONE', #1917, #11114, #9192, .T. ) ;
#5485=DIRECTION ( 'NONE',  ( 0.000000000000000000, 0.000000000000000000, 1.000000000000000000 ) ) ;
#5497=PLANE ( 'NONE',  #9761 ) ;
#5514=DIRECTION ( 'NONE',  ( -0.7071067811865504593, 0.000000000000000000, -0.7071067811865445751 ) ) ;
#5518=ORIENTED_EDGE ( 'NONE', *, *, #4393, .T. ) ;
#5520=SHAPE_REPRESENTATION_RELATIONSHIP ( 'NONE' , 'NONE' ,  #8305, #11121 ) ;
#5525=CARTESIAN_POINT ( 'NONE',  ( 9.285714285714284699, -13.00000000000000000, -3.711537444790451001 ) ) ;
#5538=EDGE_CURVE ( 'NONE', #2941, #11755, #3435, .T. ) ;
#5547=ORIENTED_EDGE ( 'NONE', *, *, #9886, .T. ) ;
#5561=VECTOR ( 'NONE', #5514, 1000.000000000000000 ) ;
#5574=CYLINDRICAL_SURFACE ( 'NONE', #11497, 4.000000000000000000 ) ;
#5588=PLANE ( 'NONE',  #1414 ) ;
#5615=DIRECTION ( 'NONE',  ( 0.000000000000000000, 1.000000000000000000, 0.000000000000000000 ) ) ;
#5617=CARTESIAN_POINT ( 'NONE',  ( -30.00000000000000000, 19.99999999999999645, 1.734723475976807094E-15 ) ) ;
#5625=AXIS2_PLACEMENT_3D ( 'NONE', #273, #11030, #5174 ) ;
#5630=PLANE ( 'NONE',  #171 ) ;
#5640=ORIENTED_EDGE ( 'NONE', *, *, #12514, .T. ) ;
#5648=ORIENTED_EDGE ( 'NONE', *, *, #333, .F. ) ;
#5664=AXIS2_PLACEMENT_3D ( 'NONE', #6399, #1691, #9592 ) ;
#5680=DIRECTION ( 'NONE',  ( 0.000000000000000000, 0.000000000000000000, 1.000000000000000000 ) ) ;
#5682=UNCERTAINTY_MEASURE_WITH_UNIT (LENGTH_MEASURE( 1.000000000000000082E-05 ), #5312, 'distance_accuracy_value', 'NONE');
#5686=CARTESIAN_POINT ( 'NONE',  ( 0.000000000000000000, -30.00000000000000000, -7.999999999999998224 ) ) ;
#5693=FACE_OUTER_BOUND ( 'NONE', #5438, .T. ) ;
#5695=VECTOR ( 'NONE', #8769, 1000.000000000000000 ) ;
#5707=CARTESIAN_POINT ( 'NONE',  ( 0.000000000000000000, 0.000000000000000000, 0.000000000000000000 ) ) ;
#5717=VERTEX_POINT ( 'NONE', #4364 ) ;
#5729=CARTESIAN_POINT ( 'NONE',  ( 14.00000000000000000, 13.00000000000000000, -6.000000000000001776 ) ) ;
#5732=AXIS2_PLACEMENT_3D ( 'NONE', #1890, #924, #12725 ) ;
#5738=CIRCLE ( 'NONE', #187, 10.00000000000000178 ) ;
#5755=DIRECTION ( 'NONE',  ( 0.000000000000000000, 1.000000000000000000, 0.000000000000000000 ) ) ;
#5758=ORIENTED_EDGE ( 'NONE', *, *, #9989, .T. ) ;
#5771=DIRECTION ( 'NONE',  ( 0.000000000000000000, 0.000000000000000000, 1.000000000000000000 ) ) ;
#5776=ORIENTED_EDGE ( 'NONE', *, *, #1275, .F. ) ;
#5779=CARTESIAN_POINT ( 'NONE',  ( -30.00000000000000000, 0.000000000000000000, 3.477184903947654954E-15 ) ) ;
#5784=MANIFOLD_SOLID_BREP ( 'Cut-Extrude1', #6004 ) ;
#5795=CARTESIAN_POINT ( 'NONE',  ( -11.83215956619923226, 30.00000000000000000, 2.000000000000000000 ) ) ;
#5837=LINE ( 'NONE', #9560, #7472 ) ;
#5840=DIRECTION ( 'NONE',  ( 0.000000000000000000, 0.000000000000000000, 1.000000000000000000 ) ) ;
#5872=DIRECTION ( 'NONE',  ( 0.000000000000000000, 0.000000000000000000, -1.000000000000000000 ) ) ;
#5875=EDGE_CURVE ( 'NONE', #3108, #4020, #7140, .T. ) ;
#5898=CARTESIAN_POINT ( 'NONE',  ( 14.00000000000000000, -30.00000000000000000, 0.000000000000000000 ) ) ;
#5916=FACE_OUTER_BOUND ( 'NONE', #1971, .T. ) ;
#5950=EDGE_LOOP ( 'NONE', ( #7629, #2240, #8747, #4359 ) ) ;
#5977=VERTEX_POINT ( 'NONE', #6860 ) ;
#5983=DIRECTION ( 'NONE',  ( -0.000000000000000000, -1.000000000000000000, -0.000000000000000000 ) ) ;
#5993=DIRECTION ( 'NONE',  ( -0.000000000000000000, -1.000000000000000000, -0.000000000000000000 ) ) ;
#5995=CARTESIAN_POINT ( 'NONE',  ( 14.00000000000000000, 30.00000000000000000, -6.000000000000000000 ) ) ;
#6004=CLOSED_SHELL ( 'NONE', ( #12141, #3464, #1287, #532, #10260, #11773, #2810, #1127, #1000, #7536, #5053, #1049, #9283, #2878, #1048, #11690, #1083, #8159, #10444, #2843, #12195, #4526, #7920, #377, #7567, #2387, #8635, #11079, #12528, #1259, #12322, #7471 ) ) ;
#6022=AXIS2_PLACEMENT_3D ( 'NONE', #2117, #6035, #6951 ) ;
#6035=DIRECTION ( 'NONE',  ( -0.000000000000000000, -0.000000000000000000, -1.000000000000000000 ) ) ;
#6084=EDGE_CURVE ( 'NONE', #6170, #5074, #8373, .T. ) ;
#6091=( NAMED_UNIT ( * ) PLANE_ANGLE_UNIT ( ) SI_UNIT ( $, .RADIAN. ) );
#6095=COLOUR_RGB ( '', 0.72549020, 0.75294118, 0.79215686) ;
#6121=AXIS2_PLACEMENT_3D ( 'NONE', #10004, #8216, #1321 ) ;
#6139=DIRECTION ( 'NONE',  ( 1.159061634649218351E-16, -0.000000000000000000, 1.000000000000000000 ) ) ;
#6142=ORIENTED_EDGE ( 'NONE', *, *, #10281, .F. ) ;
#6151=AXIS2_PLACEMENT_3D ( 'NONE', #8184, #3318, #7233 ) ;
#6154=FACE_OUTER_BOUND ( 'NONE', #237, .T. ) ;
#6158=ORIENTED_EDGE ( 'NONE', *, *, #10844, .F. ) ;
#6160=ORIENTED_EDGE ( 'NONE', *, *, #7448, .T. ) ;
#6170=VERTEX_POINT ( 'NONE', #9023 ) ;
#6210=VERTEX_POINT ( 'NONE', #4463 ) ;
#6222=VERTEX_POINT ( 'NONE', #4531 ) ;
#6234=VERTEX_POINT ( 'NONE', #7615 ) ;
#6235=CIRCLE ( 'NONE', #6660, 4.000000000000000000 ) ;
#6244=FACE_OUTER_BOUND ( 'NONE', #9443, .T. ) ;
#6256=CIRCLE ( 'NONE', #288, 2.149999999999985256 ) ;
#6257=CARTESIAN_POINT ( 'NONE',  ( 9.285714285714284699, 13.00000000000000000, -3.711537444790451001 ) ) ;
#6281=SURFACE_STYLE_USAGE ( .BOTH. , #8339 ) ;
#6305=ORIENTED_EDGE ( 'NONE', *, *, #9473, .T. ) ;
#6319=CYLINDRICAL_SURFACE ( 'NONE', #8640, 2.000000000000000888 ) ;
#6338=ORIENTED_EDGE ( 'NONE', *, *, #10201, .F. ) ;
#6355=CIRCLE ( 'NONE', #6151, 4.000000000000000000 ) ;
#6358=EDGE_LOOP ( 'NONE', ( #3846, #2214, #5199, #5158 ) ) ;
#6371=EDGE_CURVE ( 'NONE', #561, #9770, #971, .T. ) ;
#6399=CARTESIAN_POINT ( 'NONE',  ( 14.00000000000000000, 30.00000000000000000, 0.000000000000000000 ) ) ;
#6427=ORIENTED_EDGE ( 'NONE', *, *, #8803, .F. ) ;
#6428=DIRECTION ( 'NONE',  ( 1.000000000000000000, 0.000000000000000000, 0.000000000000000000 ) ) ;
#6457=CARTESIAN_POINT ( 'NONE',  ( 14.00000000000000000, -30.00000000000000000, -4.000000000000000000 ) ) ;
#6498=DIRECTION ( 'NONE',  ( -1.159061634649218351E-16, 0.000000000000000000, -1.000000000000000000 ) ) ;
#6505=LINE ( 'NONE', #6566, #12359 ) ;
#6536=DIRECTION ( 'NONE',  ( 0.000000000000000000, 1.000000000000000000, 0.000000000000000000 ) ) ;
#6566=CARTESIAN_POINT ( 'NONE',  ( -32.14999999999999147, 0.000000000000000000, 3.477184903947654954E-15 ) ) ;
#6567=VERTEX_POINT ( 'NONE', #9905 ) ;
#6575=EDGE_CURVE ( 'NONE', #6747, #3023, #5439, .T. ) ;
#6580=VECTOR ( 'NONE', #11616, 1000.000000000000000 ) ;
#6595=DIRECTION ( 'NONE',  ( 1.000000000000000000, 0.000000000000000000, 0.000000000000000000 ) ) ;
#6601=PRODUCT ( 'cover 1', 'cover 1', '', ( #7059 ) ) ;
#6602=CARTESIAN_POINT ( 'NONE',  ( 14.00000000000000000, 30.00000000000000000, 0.000000000000000000 ) ) ;
#6609=CYLINDRICAL_SURFACE ( 'NONE', #12003, 7.999999999999998224 ) ;
#6621=DIRECTION ( 'NONE',  ( 0.000000000000000000, -0.000000000000000000, 1.000000000000000000 ) ) ;
#6628=DIRECTION ( 'NONE',  ( 0.000000000000000000, -1.000000000000000000, 0.000000000000000000 ) ) ;
#6650=DIRECTION ( 'NONE',  ( 0.000000000000000000, 1.000000000000000000, 0.000000000000000000 ) ) ;
#6660=AXIS2_PLACEMENT_3D ( 'NONE', #7714, #11700, #5771 ) ;
#6663=FACE_OUTER_BOUND ( 'NONE', #4237, .T. ) ;
#6680=ORIENTED_EDGE ( 'NONE', *, *, #3070, .F. ) ;
#6708=CIRCLE ( 'NONE', #1960, 9.999999999999998224 ) ;
#6722=CARTESIAN_POINT ( 'NONE',  ( -11.83215956619923226, 30.00000000000000000, -2.000000000000000888 ) ) ;
#6741=ORIENTED_EDGE ( 'NONE', *, *, #2921, .T. ) ;
#6746=DIRECTION ( 'NONE',  ( 0.000000000000000000, 1.000000000000000000, 0.000000000000000000 ) ) ;
#6747=VERTEX_POINT ( 'NONE', #2716 ) ;
#6756=ORIENTED_EDGE ( 'NONE', *, *, #2921, .F. ) ;
#6768=LINE ( 'NONE', #2057, #12143 ) ;
#6781=CIRCLE ( 'NONE', #11705, 6.000000000000000888 ) ;
#6787=DIRECTION ( 'NONE',  ( 1.000000000000000000, 0.000000000000000000, 0.000000000000000000 ) ) ;
#6789=AXIS2_PLACEMENT_3D ( 'NONE', #7685, #785, #6787 ) ;
#6799=AXIS2_PLACEMENT_3D ( 'NONE', #11479, #6650, #5485 ) ;
#6818=DIRECTION ( 'NONE',  ( 0.000000000000000000, 1.000000000000000000, 0.000000000000000000 ) ) ;
#6849=LINE ( 'NONE', #2676, #5695 ) ;
#6854=DIRECTION ( 'NONE',  ( -0.000000000000000000, -1.000000000000000000, -0.000000000000000000 ) ) ;
#6855=CYLINDRICAL_SURFACE ( 'NONE', #10928, 6.000000000000000000 ) ;
#6859=( GEOMETRIC_REPRESENTATION_CONTEXT ( 3 ) GLOBAL_UNCERTAINTY_ASSIGNED_CONTEXT ( ( #3638 ) ) GLOBAL_UNIT_ASSIGNED_CONTEXT ( ( #10533, #10401, #7644 ) ) REPRESENTATION_CONTEXT ( 'NONE', 'WORKASPACE' ) );
#6860=CARTESIAN_POINT ( 'NONE',  ( -30.00000000000000000, 30.00000000000000000, 2.000000000000001776 ) ) ;
#6861=CYLINDRICAL_SURFACE ( 'NONE', #993, 6.000000000000000888 ) ;
#6871=FACE_OUTER_BOUND ( 'NONE', #8507, .T. ) ;
#6876=ORIENTED_EDGE ( 'NONE', *, *, #5333, .T. ) ;
#6877=DIRECTION ( 'NONE',  ( -0.000000000000000000, -1.000000000000000000, -0.000000000000000000 ) ) ;
#6917=LINE ( 'NONE', #7986, #1268 ) ;
#6936=EDGE_LOOP ( 'NONE', ( #11466, #2953, #5106, #9890 ) ) ;
#6940=DIRECTION ( 'NONE',  ( 0.000000000000000000, 0.000000000000000000, 1.000000000000000000 ) ) ;
#6951=DIRECTION ( 'NONE',  ( -1.000000000000000000, 0.000000000000000000, 0.000000000000000000 ) ) ;
#6958=ORIENTED_EDGE ( 'NONE', *, *, #7713, .T. ) ;
#6985=CIRCLE ( 'NONE', #1424, 4.000000000000000000 ) ;
#7010=VECTOR ( 'NONE', #5255, 1000.000000000000000 ) ;
#7012=EDGE_LOOP ( 'NONE', ( #6680, #2310, #10799, #3593 ) ) ;
#7018=CARTESIAN_POINT ( 'NONE',  ( 14.00000000000000000, 13.00000000000000000, 0.000000000000000000 ) ) ;
#7030=AXIS2_PLACEMENT_3D ( 'NONE', #2333, #10155, #8045 ) ;
#7033=LINE ( 'NONE', #9080, #3255 ) ;
#7035=DIRECTION ( 'NONE',  ( -0.000000000000000000, -1.000000000000000000, -0.000000000000000000 ) ) ;
#7056=ORIENTED_EDGE ( 'NONE', *, *, #10969, .F. ) ;
#7059=PRODUCT_CONTEXT ( 'NONE', #1307, 'mechanical' ) ;
#7067=CARTESIAN_POINT ( 'NONE',  ( 14.00000000000000000, 13.00000000000000000, 0.000000000000000000 ) ) ;
#7072=EDGE_LOOP ( 'NONE', ( #1523, #1252, #556, #5640 ) ) ;
#7123=CARTESIAN_POINT ( 'NONE',  ( 14.00000000000000000, -13.00000000000000000, 6.000000000000001776 ) ) ;
#7124=EDGE_LOOP ( 'NONE', ( #2299, #10420, #7182, #4208 ) ) ;
#7140=CIRCLE ( 'NONE', #751, 4.000000000000000000 ) ;
#7143=EDGE_CURVE ( 'NONE', #11779, #12600, #11427, .T. ) ;
#7145=ORIENTED_EDGE ( 'NONE', *, *, #1859, .F. ) ;
#7157=ORIENTED_EDGE ( 'NONE', *, *, #12716, .F. ) ;
#7158=FACE_OUTER_BOUND ( 'NONE', #3530, .T. ) ;
#7182=ORIENTED_EDGE ( 'NONE', *, *, #12716, .T. ) ;
#7205=VECTOR ( 'NONE', #9644, 1000.000000000000000 ) ;
#7231=DIRECTION ( 'NONE',  ( -0.000000000000000000, 1.000000000000000000, -0.000000000000000000 ) ) ;
#7232=CYLINDRICAL_SURFACE ( 'NONE', #12449, 4.000000000000000888 ) ;
#7233=DIRECTION ( 'NONE',  ( 1.000000000000000000, 0.000000000000000000, 0.000000000000000000 ) ) ;
#7237=CARTESIAN_POINT ( 'NONE',  ( 14.00000000000000000, 30.00000000000000000, 0.000000000000000000 ) ) ;
#7245=DIRECTION ( 'NONE',  ( -0.000000000000000000, -1.000000000000000000, -0.000000000000000000 ) ) ;
#7252=ORIENTED_EDGE ( 'NONE', *, *, #10627, .F. ) ;
#7260=DIRECTION ( 'NONE',  ( 0.000000000000000000, 0.000000000000000000, -1.000000000000000000 ) ) ;
#7278=CARTESIAN_POINT ( 'NONE',  ( 14.00000000000000000, -30.00000000000000000, 0.000000000000000000 ) ) ;
#7286=DIRECTION ( 'NONE',  ( -0.000000000000000000, 1.000000000000000000, 0.000000000000000000 ) ) ;
#7288=EDGE_CURVE ( 'NONE', #9393, #3905, #8967, .T. ) ;
#7296=CIRCLE ( 'NONE', #9733, 4.000000000000000000 ) ;
#7320=DIRECTION ( 'NONE',  ( -1.000000000000000000, 0.000000000000000000, 1.301042606982605074E-16 ) ) ;
#7329=EDGE_LOOP ( 'NONE', ( #2572, #1155, #3776, #3537 ) ) ;
#7347=DIRECTION ( 'NONE',  ( 0.000000000000000000, 0.000000000000000000, 1.000000000000000000 ) ) ;
#7351=CARTESIAN_POINT ( 'NONE',  ( 11.17157287525379772, 12.99999999999999822, -2.828427124746177856 ) ) ;
#7353=CARTESIAN_POINT ( 'NONE',  ( 9.285714285714284699, -3.469446951953614189E-15, -3.711537444790451001 ) ) ;
#7361=EDGE_CURVE ( 'NONE', #5977, #1661, #12672, .T. ) ;
#7369=CYLINDRICAL_SURFACE ( 'NONE', #5664, 6.000000000000000000 ) ;
#7383=EDGE_CURVE ( 'NONE', #8798, #7604, #4228, .T. ) ;
#7390=ORIENTED_EDGE ( 'NONE', *, *, #2751, .F. ) ;
#7392=DIRECTION ( 'NONE',  ( 0.000000000000000000, 0.000000000000000000, 1.000000000000000000 ) ) ;
#7404=AXIS2_PLACEMENT_3D ( 'NONE', #3968, #9041, #9934 ) ;
#7412=VECTOR ( 'NONE', #12354, 1000.000000000000000 ) ;
#7417=DIRECTION ( 'NONE',  ( 0.000000000000000000, 1.000000000000000000, 0.000000000000000000 ) ) ;
#7426=ORIENTED_EDGE ( 'NONE', *, *, #10353, .F. ) ;
#7427=CARTESIAN_POINT ( 'NONE',  ( 14.00000000000000000, 13.00000000000000000, 6.000000000000001776 ) ) ;
#7432=DIRECTION ( 'NONE',  ( 0.000000000000000000, 1.000000000000000000, 0.000000000000000000 ) ) ;
#7439=ORIENTED_EDGE ( 'NONE', *, *, #7383, .F. ) ;
#7443=CARTESIAN_POINT ( 'NONE',  ( 14.00000000000000000, 30.00000000000000000, 0.000000000000000000 ) ) ;
#7448=EDGE_CURVE ( 'NONE', #8530, #1584, #6708, .T. ) ;
#7450=ORIENTED_EDGE ( 'NONE', *, *, #8120, .F. ) ;
#7471=ADVANCED_FACE ( 'NONE', ( #1625 ), #5497, .F. ) ;
#7472=VECTOR ( 'NONE', #9749, 1000.000000000000000 ) ;
#7478=CARTESIAN_POINT ( 'NONE',  ( 11.17157287525379772, 30.00000000000000000, -2.828427124746177856 ) ) ;
#7484=VERTEX_POINT ( 'NONE', #9530 ) ;
#7492=LINE ( 'NONE', #12401, #10356 ) ;
#7493=DIRECTION ( 'NONE',  ( 0.000000000000000000, 1.000000000000000000, 0.000000000000000000 ) ) ;
#7507=CARTESIAN_POINT ( 'NONE',  ( -11.83215956619923226, 30.00000000000000000, 1.999999999999999556 ) ) ;
#7515=FILL_AREA_STYLE_COLOUR ( '', #2284 ) ;
#7528=ORIENTED_EDGE ( 'NONE', *, *, #7713, .F. ) ;
#7536=ADVANCED_FACE ( 'NONE', ( #536 ), #7369, .T. ) ;
#7554=DIRECTION ( 'NONE',  ( -0.000000000000000000, -0.000000000000000000, -1.000000000000000000 ) ) ;
#7567=ADVANCED_FACE ( 'NONE', ( #6663 ), #11428, .T. ) ;
#7569=LINE ( 'NONE', #10527, #2917 ) ;
#7579=DIRECTION ( 'NONE',  ( 0.000000000000000000, 0.000000000000000000, -1.000000000000000000 ) ) ;
#7604=VERTEX_POINT ( 'NONE', #1034 ) ;
#7615=CARTESIAN_POINT ( 'NONE',  ( -11.83215956619923226, 30.00000000000000000, -4.336808689942017736E-16 ) ) ;
#7623=EDGE_CURVE ( 'NONE', #3861, #5717, #9844, .T. ) ;
#7627=EDGE_CURVE ( 'NONE', #6234, #3861, #7923, .T. ) ;
#7629=ORIENTED_EDGE ( 'NONE', *, *, #10619, .F. ) ;
#7631=LINE ( 'NONE', #8720, #1919 ) ;
#7633=CARTESIAN_POINT ( 'NONE',  ( 11.17157287525379772, 30.00000000000000000, -2.828427124746177856 ) ) ;
#7643=ORIENTED_EDGE ( 'NONE', *, *, #10429, .T. ) ;
#7644=( NAMED_UNIT ( * ) SI_UNIT ( $, .STERADIAN. ) SOLID_ANGLE_UNIT ( ) );
#7646=ORIENTED_EDGE ( 'NONE', *, *, #1641, .T. ) ;
#7649=CARTESIAN_POINT ( 'NONE',  ( 14.00000000000000000, -12.99999999999999822, -4.000000000000000000 ) ) ;
#7655=ORIENTED_EDGE ( 'NONE', *, *, #9778, .F. ) ;
#7659=PLANE ( 'NONE',  #1498 ) ;
#7679=DIRECTION ( 'NONE',  ( 0.000000000000000000, 0.000000000000000000, 1.000000000000000000 ) ) ;
#7683=DIRECTION ( 'NONE',  ( 0.000000000000000000, 1.000000000000000000, 0.000000000000000000 ) ) ;
#7685=CARTESIAN_POINT ( 'NONE',  ( 14.00000000000000000, 30.00000000000000000, 0.000000000000000000 ) ) ;
#7713=EDGE_CURVE ( 'NONE', #1584, #6210, #4629, .T. ) ;
#7714=CARTESIAN_POINT ( 'NONE',  ( 14.00000000000000000, 12.99999999999999822, 0.000000000000000000 ) ) ;
#7731=EDGE_CURVE ( 'NONE', #11454, #2770, #5437, .T. ) ;
#7746=CARTESIAN_POINT ( 'NONE',  ( -9.860132971832690885, 30.00000000000000000, -1.666666666666667629 ) ) ;
#7771=ORIENTED_EDGE ( 'NONE', *, *, #3381, .T. ) ;
#7791=ORIENTED_EDGE ( 'NONE', *, *, #10234, .F. ) ;
#7804=DIRECTION ( 'NONE',  ( -1.159061634649218351E-16, 0.000000000000000000, -1.000000000000000000 ) ) ;
#7806=DIRECTION ( 'NONE',  ( -0.000000000000000000, -1.000000000000000000, -0.000000000000000000 ) ) ;
#7820=AXIS2_PLACEMENT_3D ( 'NONE', #991, #6621, #744 ) ;
#7826=DIRECTION ( 'NONE',  ( -0.7071067811865504593, 0.000000000000000000, -0.7071067811865445751 ) ) ;
#7831=VECTOR ( 'NONE', #7826, 1000.000000000000000 ) ;
#7842=ORIENTED_EDGE ( 'NONE', *, *, #3054, .T. ) ;
#7854=CARTESIAN_POINT ( 'NONE',  ( 14.00000000000000000, 30.00000000000000000, -6.000000000000000000 ) ) ;
#7875=DIRECTION ( 'NONE',  ( 0.000000000000000000, 0.000000000000000000, 1.000000000000000000 ) ) ;
#7920=ADVANCED_FACE ( 'NONE', ( #2336 ), #7232, .T. ) ;
#7922=CARTESIAN_POINT ( 'NONE',  ( -30.00000000000000000, -30.00000000000000000, 2.000000000000001776 ) ) ;
#7923=CIRCLE ( 'NONE', #2392, 2.000000000000000888 ) ;
#7944=EDGE_LOOP ( 'NONE', ( #7655, #7950, #8681, #4377, #11265, #6741 ) ) ;
#7950=ORIENTED_EDGE ( 'NONE', *, *, #5299, .T. ) ;
#7957=CARTESIAN_POINT ( 'NONE',  ( -11.83215956619923226, 30.00000000000000000, 1.999999999999999556 ) ) ;
#7986=CARTESIAN_POINT ( 'NONE',  ( -40.00000000000000000, -19.99999999999999645, 2.000000000000003109 ) ) ;
#7987=VECTOR ( 'NONE', #7035, 1000.000000000000000 ) ;
#7994=DIRECTION ( 'NONE',  ( -0.000000000000000000, 1.000000000000000000, -0.000000000000000000 ) ) ;
#8022=CARTESIAN_POINT ( 'NONE',  ( 9.999999999999998224, -12.99999999999999822, -6.123233995736765296E-16 ) ) ;
#8032=FACE_OUTER_BOUND ( 'NONE', #9210, .T. ) ;
#8045=DIRECTION ( 'NONE',  ( 0.000000000000000000, 0.000000000000000000, -1.000000000000000000 ) ) ;
#8082=FACE_OUTER_BOUND ( 'NONE', #5950, .T. ) ;
#8090=ORIENTED_EDGE ( 'NONE', *, *, #12719, .T. ) ;
#8117=CARTESIAN_POINT ( 'NONE',  ( 14.00000000000000000, 30.00000000000000000, -4.000000000000000000 ) ) ;
#8118=FACE_OUTER_BOUND ( 'NONE', #6358, .T. ) ;
#8120=EDGE_CURVE ( 'NONE', #7484, #803, #9754, .T. ) ;
#8142=DIRECTION ( 'NONE',  ( -0.000000000000000000, -1.000000000000000000, -0.000000000000000000 ) ) ;
#8143=ORIENTED_EDGE ( 'NONE', *, *, #8846, .T. ) ;
#8147=FILL_AREA_STYLE ('',( #10985 ) ) ;
#8159=ADVANCED_FACE ( 'NONE', ( #5916 ), #3987, .F. ) ;
#8183=CARTESIAN_POINT ( 'NONE',  ( -11.83215956619923226, 30.00000000000000000, -2.000000000000000888 ) ) ;
#8184=CARTESIAN_POINT ( 'NONE',  ( -11.83215956619923226, 30.00000000000000000, -2.000000000000000888 ) ) ;
#8216=DIRECTION ( 'NONE',  ( 0.000000000000000000, 1.000000000000000000, 0.000000000000000000 ) ) ;
#8226=CIRCLE ( 'NONE', #7404, 7.999999999999998224 ) ;
#8250=DIRECTION ( 'NONE',  ( 0.000000000000000000, 0.000000000000000000, 1.000000000000000000 ) ) ;
#8263=DIRECTION ( 'NONE',  ( 0.000000000000000000, -1.000000000000000000, 0.000000000000000000 ) ) ;
#8305=SHAPE_REPRESENTATION ( 'cover 1', ( #12422 ), #6859 ) ;
#8339=SURFACE_SIDE_STYLE ('',( #11244 ) ) ;
#8340=CYLINDRICAL_SURFACE ( 'NONE', #816, 6.000000000000000000 ) ;
#8351=CARTESIAN_POINT ( 'NONE',  ( 9.999999999999998224, 30.00000000000000000, -6.123233995736765296E-16 ) ) ;
#8356=DIRECTION ( 'NONE',  ( -1.000000000000000000, 0.000000000000000000, 1.159061634649218351E-16 ) ) ;
#8365=VERTEX_POINT ( 'NONE', #1404 ) ;
#8373=CIRCLE ( 'NONE', #10000, 6.000000000000000000 ) ;
#8379=CARTESIAN_POINT ( 'NONE',  ( -11.83215956619923226, 30.00000000000000000, -2.000000000000000888 ) ) ;
#8419=CARTESIAN_POINT ( 'NONE',  ( 14.00000000000000000, 30.00000000000000000, 0.000000000000000000 ) ) ;
#8427=AXIS2_PLACEMENT_3D ( 'NONE', #5898, #6746, #998 ) ;
#8431=FACE_OUTER_BOUND ( 'NONE', #1823, .T. ) ;
#8507=EDGE_LOOP ( 'NONE', ( #9350, #698, #6756, #5648 ) ) ;
#8530=VERTEX_POINT ( 'NONE', #3071 ) ;
#8570=CARTESIAN_POINT ( 'NONE',  ( 14.00000000000000000, 30.00000000000000000, 6.000000000000000000 ) ) ;
#8578=CARTESIAN_POINT ( 'NONE',  ( -9.860132971832690885, 30.00000000000000000, -1.666666666666667629 ) ) ;
#8582=DIRECTION ( 'NONE',  ( 1.000000000000000000, 0.000000000000000000, -1.159061634649218351E-16 ) ) ;
#8593=ORIENTED_EDGE ( 'NONE', *, *, #5283, .F. ) ;
#8604=PRESENTATION_STYLE_ASSIGNMENT (( #4751 ) ) ;
#8635=ADVANCED_FACE ( 'NONE', ( #12076 ), #11103, .T. ) ;
#8636=LINE ( 'NONE', #5795, #3138 ) ;
#8640=AXIS2_PLACEMENT_3D ( 'NONE', #8379, #3440, #10224 ) ;
#8681=ORIENTED_EDGE ( 'NONE', *, *, #8796, .T. ) ;
#8720=CARTESIAN_POINT ( 'NONE',  ( -11.83215956619923226, -30.00000000000000000, 1.999999999999999556 ) ) ;
#8722=CARTESIAN_POINT ( 'NONE',  ( 14.00000000000000000, 30.00000000000000000, 0.000000000000000000 ) ) ;
#8740=VERTEX_POINT ( 'NONE', #9344 ) ;
#8747=ORIENTED_EDGE ( 'NONE', *, *, #1607, .T. ) ;
#8757=ORIENTED_EDGE ( 'NONE', *, *, #9398, .T. ) ;
#8767=MECHANICAL_DESIGN_GEOMETRIC_PRESENTATION_REPRESENTATION('',(#2611),#9161);
#8769=DIRECTION ( 'NONE',  ( -0.000000000000000000, -1.000000000000000000, -0.000000000000000000 ) ) ;
#8770=CARTESIAN_POINT ( 'NONE',  ( 14.00000000000000000, -30.00000000000000000, 0.000000000000000000 ) ) ;
#8779=DIRECTION ( 'NONE',  ( 0.000000000000000000, 0.000000000000000000, -1.000000000000000000 ) ) ;
#8781=CYLINDRICAL_SURFACE ( 'NONE', #5732, 4.000000000000000000 ) ;
#8796=EDGE_CURVE ( 'NONE', #12099, #6234, #7492, .T. ) ;
#8798=VERTEX_POINT ( 'NONE', #10509 ) ;
#8803=EDGE_CURVE ( 'NONE', #8365, #4835, #6256, .T. ) ;
#8809=ORIENTED_EDGE ( 'NONE', *, *, #9331, .T. ) ;
#8819=ORIENTED_EDGE ( 'NONE', *, *, #6575, .F. ) ;
#8821=DIRECTION ( 'NONE',  ( -0.000000000000000000, -1.000000000000000000, -0.000000000000000000 ) ) ;
#8824=FACE_OUTER_BOUND ( 'NONE', #4576, .T. ) ;
#8834=DIRECTION ( 'NONE',  ( -0.000000000000000000, -1.000000000000000000, -0.000000000000000000 ) ) ;
#8837=DIRECTION ( 'NONE',  ( -0.000000000000000000, -0.000000000000000000, 1.000000000000000000 ) ) ;
#8842=ORIENTED_EDGE ( 'NONE', *, *, #8803, .T. ) ;
#8846=EDGE_CURVE ( 'NONE', #12605, #3108, #7296, .T. ) ;
#8851=CARTESIAN_POINT ( 'NONE',  ( 8.000000000000000000, 30.00000000000000000, -7.347880794884119736E-16 ) ) ;
#8865=EDGE_LOOP ( 'NONE', ( #11634, #5518, #2438, #10296, #10843, #829, #8090, #3839 ) ) ;
#8869=AXIS2_PLACEMENT_3D ( 'NONE', #727, #3702, #10449 ) ;
#8874=EDGE_CURVE ( 'NONE', #12600, #444, #9593, .T. ) ;
#8879=ORIENTED_EDGE ( 'NONE', *, *, #12719, .F. ) ;
#8922=VERTEX_POINT ( 'NONE', #9908 ) ;
#8923=CIRCLE ( 'NONE', #898, 4.000000000000000000 ) ;
#8967=LINE ( 'NONE', #4987, #10800 ) ;
#8981=LINE ( 'NONE', #12680, #12339 ) ;
#8987=EDGE_CURVE ( 'NONE', #6567, #9408, #2073, .T. ) ;
#8990=ORIENTED_EDGE ( 'NONE', *, *, #5405, .T. ) ;
#8998=ORIENTED_EDGE ( 'NONE', *, *, #12320, .F. ) ;
#9012=CIRCLE ( 'NONE', #9406, 4.000000000000000000 ) ;
#9013=EDGE_CURVE ( 'NONE', #6234, #9770, #974, .T. ) ;
#9023=CARTESIAN_POINT ( 'NONE',  ( 8.000000000000000000, 30.00000000000000000, -7.347880794884119736E-16 ) ) ;
#9041=DIRECTION ( 'NONE',  ( -0.000000000000000000, -1.000000000000000000, -0.000000000000000000 ) ) ;
#9043=ORIENTED_EDGE ( 'NONE', *, *, #9158, .F. ) ;
#9074=CARTESIAN_POINT ( 'NONE',  ( -40.00000000000000000, 30.00000000000000000, 2.000000000000003109 ) ) ;
#9080=CARTESIAN_POINT ( 'NONE',  ( 14.00000000000000000, 30.00000000000000000, 4.000000000000000000 ) ) ;
#9085=CIRCLE ( 'NONE', #10945, 9.999999999999998224 ) ;
#9113=FACE_OUTER_BOUND ( 'NONE', #8865, .T. ) ;
#9116=VECTOR ( 'NONE', #8837, 1000.000000000000000 ) ;
#9120=VERTEX_POINT ( 'NONE', #3376 ) ;
#9125=CARTESIAN_POINT ( 'NONE',  ( -40.00000000000000000, -19.99999999999999645, 2.831145448779744488E-15 ) ) ;
#9158=EDGE_CURVE ( 'NONE', #10545, #1458, #6355, .T. ) ;
#9161=( GEOMETRIC_REPRESENTATION_CONTEXT ( 3 ) GLOBAL_UNCERTAINTY_ASSIGNED_CONTEXT ( ( #5682 ) ) GLOBAL_UNIT_ASSIGNED_CONTEXT ( ( #5312, #6091, #5130 ) ) REPRESENTATION_CONTEXT ( 'NONE', 'WORKASPACE' ) );
#9168=FACE_OUTER_BOUND ( 'NONE', #2183, .T. ) ;
#9192=CIRCLE ( 'NONE', #12475, 6.000000000000000888 ) ;
#9210=EDGE_LOOP ( 'NONE', ( #3582, #2391, #12417, #2600 ) ) ;
#9260=CARTESIAN_POINT ( 'NONE',  ( -40.00000000000000000, 30.00000000000000000, 2.000000000000003109 ) ) ;
#9270=ORIENTED_EDGE ( 'NONE', *, *, #1275, .T. ) ;
#9277=CARTESIAN_POINT ( 'NONE',  ( -30.00000000000000000, -30.00000000000000000, 2.831145448779744488E-15 ) ) ;
#9283=ADVANCED_FACE ( 'NONE', ( #2465 ), #5415, .T. ) ;
#9286=DIRECTION ( 'NONE',  ( -1.000000000000000000, 0.000000000000000000, 2.017120320903271344E-16 ) ) ;
#9293=CARTESIAN_POINT ( 'NONE',  ( 0.000000000000000000, 30.00000000000000000, 0.000000000000000000 ) ) ;
#9297=LINE ( 'NONE', #4488, #7010 ) ;
#9306=CARTESIAN_POINT ( 'NONE',  ( 14.00000000000000000, 30.00000000000000000, -4.000000000000000000 ) ) ;
#9308=VERTEX_POINT ( 'NONE', #12386 ) ;
#9312=DIRECTION ( 'NONE',  ( 0.000000000000000000, 0.000000000000000000, -1.000000000000000000 ) ) ;
#9320=CARTESIAN_POINT ( 'NONE',  ( -30.00000000000000000, 0.000000000000000000, 2.000000000000001776 ) ) ;
#9328=DIRECTION ( 'NONE',  ( 0.7071067811865504593, 0.000000000000000000, 0.7071067811865445751 ) ) ;
#9331=EDGE_CURVE ( 'NONE', #9308, #412, #707, .T. ) ;
#9344=CARTESIAN_POINT ( 'NONE',  ( 11.17157287525379772, 30.00000000000000000, -2.828427124746177856 ) ) ;
#9350=ORIENTED_EDGE ( 'NONE', *, *, #3381, .F. ) ;
#9358=LINE ( 'NONE', #7507, #7412 ) ;
#9369=DIRECTION ( 'NONE',  ( -0.000000000000000000, -1.000000000000000000, -0.000000000000000000 ) ) ;
#9390=LINE ( 'NONE', #8570, #7205 ) ;
#9393=VERTEX_POINT ( 'NONE', #12575 ) ;
#9398=EDGE_CURVE ( 'NONE', #11114, #3023, #1926, .T. ) ;
#9402=CARTESIAN_POINT ( 'NONE',  ( -30.00000000000000000, 0.000000000000000000, 2.185182530847200403E-15 ) ) ;
#9406=AXIS2_PLACEMENT_3D ( 'NONE', #8722, #5755, #7875 ) ;
#9408=VERTEX_POINT ( 'NONE', #5729 ) ;
#9422=ORIENTED_EDGE ( 'NONE', *, *, #9569, .F. ) ;
#9427=CIRCLE ( 'NONE', #3897, 9.999999999999998224 ) ;
#9443=EDGE_LOOP ( 'NONE', ( #1200, #10827, #12435, #4574 ) ) ;
#9473=EDGE_CURVE ( 'NONE', #8922, #444, #6768, .T. ) ;
#9490=ORIENTED_EDGE ( 'NONE', *, *, #5283, .T. ) ;
#9498=DIRECTION ( 'NONE',  ( -1.159061634649218351E-16, 0.000000000000000000, -1.000000000000000000 ) ) ;
#9508=DIRECTION ( 'NONE',  ( 0.000000000000000000, -0.000000000000000000, 1.000000000000000000 ) ) ;
#9528=DIRECTION ( 'NONE',  ( -1.000000000000000000, 0.000000000000000000, 1.159061634649218351E-16 ) ) ;
#9530=CARTESIAN_POINT ( 'NONE',  ( 9.999999999999998224, 12.99999999999999822, -6.123233995736765296E-16 ) ) ;
#9551=VERTEX_POINT ( 'NONE', #3302 ) ;
#9560=CARTESIAN_POINT ( 'NONE',  ( 14.00000000000000000, 30.00000000000000000, -4.000000000000000000 ) ) ;
#9569=EDGE_CURVE ( 'NONE', #2770, #6747, #3103, .T. ) ;
#9592=DIRECTION ( 'NONE',  ( 0.000000000000000000, 0.000000000000000000, -1.000000000000000000 ) ) ;
#9593=LINE ( 'NONE', #11615, #10770 ) ;
#9599=ORIENTED_EDGE ( 'NONE', *, *, #5538, .T. ) ;
#9639=CARTESIAN_POINT ( 'NONE',  ( 14.00000000000000000, 30.00000000000000000, 0.000000000000000000 ) ) ;
#9644=DIRECTION ( 'NONE',  ( -0.000000000000000000, -1.000000000000000000, -0.000000000000000000 ) ) ;
#9653=CARTESIAN_POINT ( 'NONE',  ( 9.757359312880696578, -30.00000000000000000, -4.242640687119267007 ) ) ;
#9658=VECTOR ( 'NONE', #5056, 1000.000000000000000 ) ;
#9689=EDGE_CURVE ( 'NONE', #3082, #4835, #6505, .T. ) ;
#9728=CARTESIAN_POINT ( 'NONE',  ( 0.000000000000000000, 30.00000000000000000, 0.000000000000000000 ) ) ;
#9733=AXIS2_PLACEMENT_3D ( 'NONE', #11492, #6536, #5680 ) ;
#9738=DIRECTION ( 'NONE',  ( -0.7071067811865504593, 0.000000000000000000, -0.7071067811865445751 ) ) ;
#9739=ORIENTED_EDGE ( 'NONE', *, *, #333, .T. ) ;
#9749=DIRECTION ( 'NONE',  ( -0.000000000000000000, -1.000000000000000000, -0.000000000000000000 ) ) ;
#9754=CIRCLE ( 'NONE', #4216, 4.000000000000000000 ) ;
#9759=DIRECTION ( 'NONE',  ( -1.000000000000000000, 0.000000000000000000, 0.000000000000000000 ) ) ;
#9761=AXIS2_PLACEMENT_3D ( 'NONE', #12399, #7432, #10307 ) ;
#9770=VERTEX_POINT ( 'NONE', #12434 ) ;
#9778=EDGE_CURVE ( 'NONE', #9551, #2818, #9297, .T. ) ;
#9802=CYLINDRICAL_SURFACE ( 'NONE', #7820, 10.00000000000000178 ) ;
#9806=VECTOR ( 'NONE', #9312, 1000.000000000000000 ) ;
#9844=LINE ( 'NONE', #7746, #729 ) ;
#9881=EDGE_CURVE ( 'NONE', #5977, #10545, #9358, .T. ) ;
#9882=ORIENTED_EDGE ( 'NONE', *, *, #10009, .F. ) ;
#9886=EDGE_CURVE ( 'NONE', #711, #412, #10395, .T. ) ;
#9890=ORIENTED_EDGE ( 'NONE', *, *, #7623, .T. ) ;
#9905=CARTESIAN_POINT ( 'NONE',  ( 14.00000000000000000, 30.00000000000000000, -6.000000000000000000 ) ) ;
#9908=CARTESIAN_POINT ( 'NONE',  ( 9.757359312880696578, -13.00000000000000000, -4.242640687119267895 ) ) ;
#9934=DIRECTION ( 'NONE',  ( 1.000000000000000000, 0.000000000000000000, 0.000000000000000000 ) ) ;
#9984=EDGE_CURVE ( 'NONE', #4020, #8922, #7569, .T. ) ;
#9985=CARTESIAN_POINT ( 'NONE',  ( -30.00000000000000000, 19.99999999999999645, 2.000000000000001776 ) ) ;
#9989=EDGE_CURVE ( 'NONE', #8740, #9308, #4863, .T. ) ;
#9990=ORIENTED_EDGE ( 'NONE', *, *, #4552, .T. ) ;
#10000=AXIS2_PLACEMENT_3D ( 'NONE', #12071, #3197, #3262 ) ;
#10004=CARTESIAN_POINT ( 'NONE',  ( -11.83215956619923226, -30.00000000000000000, -2.000000000000000888 ) ) ;
#10009=EDGE_CURVE ( 'NONE', #1458, #7604, #2157, .T. ) ;
#10024=LINE ( 'NONE', #1217, #2033 ) ;
#10027=CARTESIAN_POINT ( 'NONE',  ( -29.99999999999999289, 30.00000000000000000, 1.672083814130525448E-15 ) ) ;
#10040=DIRECTION ( 'NONE',  ( 0.000000000000000000, 0.000000000000000000, 1.000000000000000000 ) ) ;
#10065=ORIENTED_EDGE ( 'NONE', *, *, #1820, .F. ) ;
#10100=DIRECTION ( 'NONE',  ( 0.000000000000000000, 0.000000000000000000, 1.000000000000000000 ) ) ;
#10106=AXIS2_PLACEMENT_3D ( 'NONE', #5159, #12056, #3245 ) ;
#10150=ORIENTED_EDGE ( 'NONE', *, *, #2352, .T. ) ;
#10155=DIRECTION ( 'NONE',  ( -0.000000000000000000, -1.000000000000000000, -0.000000000000000000 ) ) ;
#10157=DIRECTION ( 'NONE',  ( -0.000000000000000000, -1.000000000000000000, -0.000000000000000000 ) ) ;
#10177=ORIENTED_EDGE ( 'NONE', *, *, #7627, .F. ) ;
#10187=CARTESIAN_POINT ( 'NONE',  ( 14.00000000000000000, 30.00000000000000000, 0.000000000000000000 ) ) ;
#10189=DIRECTION ( 'NONE',  ( -1.000000000000000000, 0.000000000000000000, 1.159061634649218351E-16 ) ) ;
#10201=EDGE_CURVE ( 'NONE', #6567, #9308, #2042, .T. ) ;
#10203=VECTOR ( 'NONE', #2805, 1000.000000000000000 ) ;
#10215=DIRECTION ( 'NONE',  ( 0.000000000000000000, 0.000000000000000000, 1.000000000000000000 ) ) ;
#10224=DIRECTION ( 'NONE',  ( 0.000000000000000000, 0.000000000000000000, -1.000000000000000000 ) ) ;
#10227=ORIENTED_EDGE ( 'NONE', *, *, #3496, .T. ) ;
#10234=EDGE_CURVE ( 'NONE', #4020, #12600, #661, .T. ) ;
#10260=ADVANCED_FACE ( 'NONE', ( #10636 ), #12524, .T. ) ;
#10281=EDGE_CURVE ( 'NONE', #3923, #6222, #6985, .T. ) ;
#10287=DIRECTION ( 'NONE',  ( -1.000000000000000000, 0.000000000000000000, 2.017120320903271344E-16 ) ) ;
#10296=ORIENTED_EDGE ( 'NONE', *, *, #4328, .F. ) ;
#10307=DIRECTION ( 'NONE',  ( 0.000000000000000000, -0.000000000000000000, 1.000000000000000000 ) ) ;
#10316=ORIENTED_EDGE ( 'NONE', *, *, #8874, .F. ) ;
#10317=ORIENTED_EDGE ( 'NONE', *, *, #9331, .F. ) ;
#10327=EDGE_LOOP ( 'NONE', ( #11357, #8990, #7450, #7056 ) ) ;
#10335=FILL_AREA_STYLE ('',( #7515 ) ) ;
#10353=EDGE_CURVE ( 'NONE', #3861, #9120, #9427, .T. ) ;
#10356=VECTOR ( 'NONE', #8582, 1000.000000000000000 ) ;
#10376=CARTESIAN_POINT ( 'NONE',  ( 14.00000000000000000, 30.00000000000000000, 0.000000000000000000 ) ) ;
#10395=LINE ( 'NONE', #1580, #5561 ) ;
#10401=( NAMED_UNIT ( * ) PLANE_ANGLE_UNIT ( ) SI_UNIT ( $, .RADIAN. ) );
#10408=LINE ( 'NONE', #1594, #9806 ) ;
#10420=ORIENTED_EDGE ( 'NONE', *, *, #10627, .T. ) ;
#10429=EDGE_CURVE ( 'NONE', #12605, #6210, #12717, .T. ) ;
#10430=CARTESIAN_POINT ( 'NONE',  ( 9.757359312880696578, 30.00000000000000000, -4.242640687119267007 ) ) ;
#10433=AXIS2_PLACEMENT_3D ( 'NONE', #3789, #1910, #11703 ) ;
#10444=ADVANCED_FACE ( 'NONE', ( #1293 ), #6319, .F. ) ;
#10449=DIRECTION ( 'NONE',  ( 0.000000000000000000, 0.000000000000000000, 1.000000000000000000 ) ) ;
#10462=ORIENTED_EDGE ( 'NONE', *, *, #11872, .T. ) ;
#10469=AXIS2_PLACEMENT_3D ( 'NONE', #7478, #12315, #9328 ) ;
#10509=CARTESIAN_POINT ( 'NONE',  ( -11.83215956619923226, -30.00000000000000000, 2.000000000000000000 ) ) ;
#10527=CARTESIAN_POINT ( 'NONE',  ( 11.17157287525379772, -12.99999999999999822, -2.828427124746177856 ) ) ;
#10532=VERTEX_POINT ( 'NONE', #8117 ) ;
#10533=( LENGTH_UNIT ( ) NAMED_UNIT ( * ) SI_UNIT ( .MILLI., .METRE. ) );
#10540=CARTESIAN_POINT ( 'NONE',  ( -27.85000000000000497, 2.632990618166804305E-16, 2.000000000000001332 ) ) ;
#10545=VERTEX_POINT ( 'NONE', #3320 ) ;
#10566=DIRECTION ( 'NONE',  ( 0.000000000000000000, 0.000000000000000000, 1.000000000000000000 ) ) ;
#10592=ORIENTED_EDGE ( 'NONE', *, *, #3514, .T. ) ;
#10593=CARTESIAN_POINT ( 'NONE',  ( 14.00000000000000000, -13.00000000000000000, -6.000000000000001776 ) ) ;
#10608=ORIENTED_EDGE ( 'NONE', *, *, #8120, .T. ) ;
#10619=EDGE_CURVE ( 'NONE', #1917, #6747, #9390, .T. ) ;
#10625=CIRCLE ( 'NONE', #12496, 10.00000000000000178 ) ;
#10627=EDGE_CURVE ( 'NONE', #6222, #10532, #3909, .T. ) ;
#10636=FACE_OUTER_BOUND ( 'NONE', #1586, .T. ) ;
#10639=ORIENTED_EDGE ( 'NONE', *, *, #1820, .T. ) ;
#10641=CARTESIAN_POINT ( 'NONE',  ( -30.00000000000000000, 30.00000000000000000, 0.000000000000000000 ) ) ;
#10651=ORIENTED_EDGE ( 'NONE', *, *, #9886, .F. ) ;
#10679=DIRECTION ( 'NONE',  ( -0.000000000000000000, -1.000000000000000000, -0.000000000000000000 ) ) ;
#10736=EDGE_LOOP ( 'NONE', ( #7791, #475, #6305, #10316 ) ) ;
#10738=VECTOR ( 'NONE', #464, 1000.000000000000000 ) ;
#10770=VECTOR ( 'NONE', #2809, 1000.000000000000000 ) ;
#10779=AXIS2_PLACEMENT_3D ( 'NONE', #8770, #7683, #77 ) ;
#10788=CARTESIAN_POINT ( 'NONE',  ( -32.14999999999999147, 0.000000000000000000, 2.000000000000002220 ) ) ;
#10792=AXIS2_PLACEMENT_3D ( 'NONE', #9639, #1924, #11791 ) ;
#10797=FACE_OUTER_BOUND ( 'NONE', #7072, .T. ) ;
#10799=ORIENTED_EDGE ( 'NONE', *, *, #10234, .T. ) ;
#10800=VECTOR ( 'NONE', #11884, 1000.000000000000000 ) ;
#10827=ORIENTED_EDGE ( 'NONE', *, *, #4198, .T. ) ;
#10843=ORIENTED_EDGE ( 'NONE', *, *, #5538, .F. ) ;
#10844=EDGE_CURVE ( 'NONE', #9393, #303, #11538, .T. ) ;
#10928=AXIS2_PLACEMENT_3D ( 'NONE', #4915, #8834, #12063 ) ;
#10931=CARTESIAN_POINT ( 'NONE',  ( 0.000000000000000000, 30.00000000000000000, 0.000000000000000000 ) ) ;
#10933=CARTESIAN_POINT ( 'NONE',  ( 14.00000000000000000, 12.99999999999999822, 0.000000000000000000 ) ) ;
#10936=PRODUCT_DEFINITION_CONTEXT ( 'detailed design', #4366, 'design' ) ;
#10944=CARTESIAN_POINT ( 'NONE',  ( 14.00000000000000000, -30.00000000000000000, 0.000000000000000000 ) ) ;
#10945=AXIS2_PLACEMENT_3D ( 'NONE', #12185, #5343, #7347 ) ;
#10948=DIRECTION ( 'NONE',  ( 0.000000000000000000, 1.000000000000000000, 0.000000000000000000 ) ) ;
#10965=CARTESIAN_POINT ( 'NONE',  ( 0.000000000000000000, -30.00000000000000000, 0.000000000000000000 ) ) ;
#10969=EDGE_CURVE ( 'NONE', #3923, #7484, #10024, .T. ) ;
#10983=ORIENTED_EDGE ( 'NONE', *, *, #11688, .T. ) ;
#10985=FILL_AREA_STYLE_COLOUR ( '', #6095 ) ;
#10987=LINE ( 'NONE', #1385, #12506 ) ;
#11017=CYLINDRICAL_SURFACE ( 'NONE', #7030, 4.000000000000000000 ) ;
#11019=AXIS2_PLACEMENT_3D ( 'NONE', #10376, #722, #2745 ) ;
#11030=DIRECTION ( 'NONE',  ( -0.000000000000000000, -1.000000000000000000, -0.000000000000000000 ) ) ;
#11048=ORIENTED_EDGE ( 'NONE', *, *, #11688, .F. ) ;
#11060=CIRCLE ( 'NONE', #768, 9.999999999999998224 ) ;
#11066=CYLINDRICAL_SURFACE ( 'NONE', #4513, 9.999999999999998224 ) ;
#11079=ADVANCED_FACE ( 'NONE', ( #6871 ), #9802, .T. ) ;
#11103=CYLINDRICAL_SURFACE ( 'NONE', #1112, 10.00000000000000178 ) ;
#11106=ORIENTED_EDGE ( 'NONE', *, *, #9881, .T. ) ;
#11114=VERTEX_POINT ( 'NONE', #10593 ) ;
#11121=ADVANCED_BREP_SHAPE_REPRESENTATION ( '', ( #5784, #12422 ), #6859 ) ;
#11144=CYLINDRICAL_SURFACE ( 'NONE', #10106, 2.149999999999992362 ) ;
#11159=ORIENTED_EDGE ( 'NONE', *, *, #5020, .T. ) ;
#11163=DIRECTION ( 'NONE',  ( 1.000000000000000000, 0.000000000000000000, 0.000000000000000000 ) ) ;
#11180=CYLINDRICAL_SURFACE ( 'NONE', #5109, 4.000000000000000000 ) ;
#11200=DIRECTION ( 'NONE',  ( 1.000000000000000000, 0.000000000000000000, 0.000000000000000000 ) ) ;
#11212=DIRECTION ( 'NONE',  ( 1.000000000000000000, 0.000000000000000000, 0.000000000000000000 ) ) ;
#11218=DIRECTION ( 'NONE',  ( 0.000000000000000000, 0.000000000000000000, -1.000000000000000000 ) ) ;
#11225=EDGE_CURVE ( 'NONE', #6170, #9393, #4931, .T. ) ;
#11244=SURFACE_STYLE_FILL_AREA ( #8147 ) ;
#11259=CARTESIAN_POINT ( 'NONE',  ( 14.00000000000000000, -12.99999999999999822, 4.000000000000000000 ) ) ;
#11265=ORIENTED_EDGE ( 'NONE', *, *, #6371, .F. ) ;
#11293=EDGE_CURVE ( 'NONE', #3082, #4276, #4765, .T. ) ;
#11309=AXIS2_PLACEMENT_3D ( 'NONE', #6602, #11493, #1817 ) ;
#11337=DIRECTION ( 'NONE',  ( -0.000000000000000000, -0.000000000000000000, -1.000000000000000000 ) ) ;
#11357=ORIENTED_EDGE ( 'NONE', *, *, #10281, .T. ) ;
#11370=ORIENTED_EDGE ( 'NONE', *, *, #10009, .T. ) ;
#11377=EDGE_CURVE ( 'NONE', #11114, #8922, #234, .T. ) ;
#11415=ORIENTED_EDGE ( 'NONE', *, *, #10429, .F. ) ;
#11421=ORIENTED_EDGE ( 'NONE', *, *, #9689, .F. ) ;
#11427=CIRCLE ( 'NONE', #4641, 4.000000000000000000 ) ;
#11428=PLANE ( 'NONE',  #11019 ) ;
#11436=ORIENTED_EDGE ( 'NONE', *, *, #5020, .F. ) ;
#11439=DIRECTION ( 'NONE',  ( 0.7071067811865504593, 0.000000000000000000, 0.7071067811865445751 ) ) ;
#11442=CARTESIAN_POINT ( 'NONE',  ( 14.00000000000000000, -30.00000000000000000, 0.000000000000000000 ) ) ;
#11445=ORIENTED_EDGE ( 'NONE', *, *, #8987, .T. ) ;
#11452=( NAMED_UNIT ( * ) PLANE_ANGLE_UNIT ( ) SI_UNIT ( $, .RADIAN. ) );
#11454=VERTEX_POINT ( 'NONE', #5686 ) ;
#11459=ORIENTED_EDGE ( 'NONE', *, *, #4328, .T. ) ;
#11463=CIRCLE ( 'NONE', #1790, 7.999999999999998224 ) ;
#11466=ORIENTED_EDGE ( 'NONE', *, *, #4483, .F. ) ;
#11479=CARTESIAN_POINT ( 'NONE',  ( 14.00000000000000000, 30.00000000000000000, 0.000000000000000000 ) ) ;
#11492=CARTESIAN_POINT ( 'NONE',  ( 14.00000000000000000, -12.99999999999999822, 0.000000000000000000 ) ) ;
#11493=DIRECTION ( 'NONE',  ( -0.000000000000000000, -1.000000000000000000, -0.000000000000000000 ) ) ;
#11497=AXIS2_PLACEMENT_3D ( 'NONE', #7443, #4549, #12535 ) ;
#11515=ORIENTED_EDGE ( 'NONE', *, *, #8846, .F. ) ;
#11522=CYLINDRICAL_SURFACE ( 'NONE', #2461, 4.000000000000000000 ) ;
#11538=CIRCLE ( 'NONE', #12154, 6.000000000000000888 ) ;
#11539=VECTOR ( 'NONE', #1283, 1000.000000000000000 ) ;
#11565=DIRECTION ( 'NONE',  ( 1.000000000000000000, 0.000000000000000000, -1.159061634649218351E-16 ) ) ;
#11571=EDGE_CURVE ( 'NONE', #2818, #235, #6917, .T. ) ;
#11580=AXIS2_PLACEMENT_3D ( 'NONE', #9260, #3488, #10215 ) ;
#11593=CARTESIAN_POINT ( 'NONE',  ( 14.00000000000000000, -13.00000000000000000, 0.000000000000000000 ) ) ;
#11615=CARTESIAN_POINT ( 'NONE',  ( 11.17157287525379772, -30.00000000000000000, -2.828427124746177856 ) ) ;
#11616=DIRECTION ( 'NONE',  ( -0.000000000000000000, -1.000000000000000000, -0.000000000000000000 ) ) ;
#11617=UNCERTAINTY_MEASURE_WITH_UNIT (LENGTH_MEASURE( 1.000000000000000082E-05 ), #12424, 'distance_accuracy_value', 'NONE');
#11626=DIRECTION ( 'NONE',  ( -0.7071067811865445751, 0.000000000000000000, 0.7071067811865504593 ) ) ;
#11634=ORIENTED_EDGE ( 'NONE', *, *, #2184, .F. ) ;
#11669=CIRCLE ( 'NONE', #2417, 4.000000000000000000 ) ;
#11672=CYLINDRICAL_SURFACE ( 'NONE', #42, 7.999999999999998224 ) ;
#11677=DIRECTION ( 'NONE',  ( -0.000000000000000000, -1.000000000000000000, -0.000000000000000000 ) ) ;
#11679=AXIS2_PLACEMENT_3D ( 'NONE', #7067, #4164, #358 ) ;
#11688=EDGE_CURVE ( 'NONE', #303, #9408, #1686, .T. ) ;
#11690=ADVANCED_FACE ( 'NONE', ( #8118 ), #6855, .T. ) ;
#11695=VERTEX_POINT ( 'NONE', #395 ) ;
#11700=DIRECTION ( 'NONE',  ( 0.000000000000000000, 1.000000000000000000, 0.000000000000000000 ) ) ;
#11703=DIRECTION ( 'NONE',  ( 0.000000000000000000, 0.000000000000000000, -1.000000000000000000 ) ) ;
#11705=AXIS2_PLACEMENT_3D ( 'NONE', #2901, #6818, #6940 ) ;
#11735=CARTESIAN_POINT ( 'NONE',  ( 0.000000000000000000, 30.00000000000000000, -9.999999999999998224 ) ) ;
#11741=STYLED_ITEM ( 'NONE', ( #8604 ), #11121 ) ;
#11755=VERTEX_POINT ( 'NONE', #6257 ) ;
#11773=ADVANCED_FACE ( 'NONE', ( #1357 ), #12129, .T. ) ;
#11779=VERTEX_POINT ( 'NONE', #6457 ) ;
#11783=CYLINDRICAL_SURFACE ( 'NONE', #1701, 2.149999999999992362 ) ;
#11791=DIRECTION ( 'NONE',  ( 0.000000000000000000, 0.000000000000000000, -1.000000000000000000 ) ) ;
#11809=CARTESIAN_POINT ( 'NONE',  ( 0.000000000000000000, 30.00000000000000000, 0.000000000000000000 ) ) ;
#11827=DIRECTION ( 'NONE',  ( -0.000000000000000000, -1.000000000000000000, -0.000000000000000000 ) ) ;
#11863=FACE_OUTER_BOUND ( 'NONE', #7124, .T. ) ;
#11868=DIRECTION ( 'NONE',  ( -0.000000000000000000, -1.000000000000000000, -0.000000000000000000 ) ) ;
#11872=EDGE_CURVE ( 'NONE', #10545, #8798, #8636, .T. ) ;
#11883=EDGE_LOOP ( 'NONE', ( #617, #1016, #9599, #5188 ) ) ;
#11884=DIRECTION ( 'NONE',  ( -0.000000000000000000, -1.000000000000000000, -0.000000000000000000 ) ) ;
#11908=EDGE_LOOP ( 'NONE', ( #11436, #3092, #158, #399, #4478, #29 ) ) ;
#11915=AXIS2_PLACEMENT_3D ( 'NONE', #2574, #6628, #2509 ) ;
#11917=ORIENTED_EDGE ( 'NONE', *, *, #3070, .T. ) ;
#11936=AXIS2_PLACEMENT_3D ( 'NONE', #4246, #3174, #2258 ) ;
#11973=ORIENTED_EDGE ( 'NONE', *, *, #5470, .F. ) ;
#11980=DIRECTION ( 'NONE',  ( 0.000000000000000000, 0.000000000000000000, -1.000000000000000000 ) ) ;
#12003=AXIS2_PLACEMENT_3D ( 'NONE', #9728, #2943, #8779 ) ;
#12020=SHAPE_DEFINITION_REPRESENTATION ( #4644, #8305 ) ;
#12022=ORIENTED_EDGE ( 'NONE', *, *, #10201, .T. ) ;
#12029=CARTESIAN_POINT ( 'NONE',  ( 14.00000000000000000, 30.00000000000000000, 0.000000000000000000 ) ) ;
#12030=CARTESIAN_POINT ( 'NONE',  ( 0.000000000000000000, 30.00000000000000000, -7.999999999999998224 ) ) ;
#12056=DIRECTION ( 'NONE',  ( -0.000000000000000000, -0.000000000000000000, -1.000000000000000000 ) ) ;
#12058=LINE ( 'NONE', #9074, #11539 ) ;
#12063=DIRECTION ( 'NONE',  ( 0.000000000000000000, 0.000000000000000000, -1.000000000000000000 ) ) ;
#12071=CARTESIAN_POINT ( 'NONE',  ( 14.00000000000000000, 30.00000000000000000, 0.000000000000000000 ) ) ;
#12075=CIRCLE ( 'NONE', #1575, 6.000000000000000888 ) ;
#12076=FACE_OUTER_BOUND ( 'NONE', #7329, .T. ) ;
#12079=ORIENTED_EDGE ( 'NONE', *, *, #5231, .F. ) ;
#12099=VERTEX_POINT ( 'NONE', #10027 ) ;
#12100=CIRCLE ( 'NONE', #11679, 6.000000000000000888 ) ;
#12125=CARTESIAN_POINT ( 'NONE',  ( 14.00000000000000000, -13.00000000000000000, 0.000000000000000000 ) ) ;
#12129=CYLINDRICAL_SURFACE ( 'NONE', #1885, 6.000000000000000000 ) ;
#12141=ADVANCED_FACE ( 'NONE', ( #7158 ), #11144, .F. ) ;
#12142=DIRECTION ( 'NONE',  ( 1.000000000000000000, 0.000000000000000000, 0.000000000000000000 ) ) ;
#12143=VECTOR ( 'NONE', #5983, 1000.000000000000000 ) ;
#12154=AXIS2_PLACEMENT_3D ( 'NONE', #4185, #4249, #12357 ) ;
#12185=CARTESIAN_POINT ( 'NONE',  ( 0.000000000000000000, -12.99999999999999822, 0.000000000000000000 ) ) ;
#12195=ADVANCED_FACE ( 'NONE', ( #6244 ), #12310, .T. ) ;
#12196=DIRECTION ( 'NONE',  ( -0.000000000000000000, -1.000000000000000000, -0.000000000000000000 ) ) ;
#12203=EDGE_CURVE ( 'NONE', #4276, #3082, #1895, .T. ) ;
#12238=EDGE_CURVE ( 'NONE', #2941, #4489, #9085, .T. ) ;
#12272=ORIENTED_EDGE ( 'NONE', *, *, #8874, .T. ) ;
#12296=DIRECTION ( 'NONE',  ( -0.000000000000000000, -1.000000000000000000, -0.000000000000000000 ) ) ;
#12310=PLANE ( 'NONE',  #11580 ) ;
#12315=DIRECTION ( 'NONE',  ( -0.7071067811865445751, 0.000000000000000000, 0.7071067811865504593 ) ) ;
#12320=EDGE_CURVE ( 'NONE', #3023, #444, #2537, .T. ) ;
#12322=ADVANCED_FACE ( 'NONE', ( #8431 ), #7659, .T. ) ;
#12335=CIRCLE ( 'NONE', #4714, 6.000000000000000888 ) ;
#12338=ORIENTED_EDGE ( 'NONE', *, *, #4483, .T. ) ;
#12339=VECTOR ( 'NONE', #6877, 1000.000000000000000 ) ;
#12343=ORIENTED_EDGE ( 'NONE', *, *, #1942, .T. ) ;
#12353=DIRECTION ( 'NONE',  ( 0.000000000000000000, 1.000000000000000000, 0.000000000000000000 ) ) ;
#12354=DIRECTION ( 'NONE',  ( 1.000000000000000000, 0.000000000000000000, -1.159061634649218351E-16 ) ) ;
#12357=DIRECTION ( 'NONE',  ( 0.000000000000000000, 0.000000000000000000, 1.000000000000000000 ) ) ;
#12359=VECTOR ( 'NONE', #11337, 1000.000000000000000 ) ;
#12364=( NAMED_UNIT ( * ) SI_UNIT ( $, .STERADIAN. ) SOLID_ANGLE_UNIT ( ) );
#12386=CARTESIAN_POINT ( 'NONE',  ( 9.757359312880696578, 30.00000000000000000, -4.242640687119267007 ) ) ;
#12399=CARTESIAN_POINT ( 'NONE',  ( 14.00000000000000000, 13.00000000000000000, 0.000000000000000000 ) ) ;
#12401=CARTESIAN_POINT ( 'NONE',  ( -11.83215956619923226, 30.00000000000000000, -4.336808689942017736E-16 ) ) ;
#12417=ORIENTED_EDGE ( 'NONE', *, *, #2850, .F. ) ;
#12422=AXIS2_PLACEMENT_3D ( 'NONE', #5707, #7392, #6428 ) ;
#12424=( LENGTH_UNIT ( ) NAMED_UNIT ( * ) SI_UNIT ( .MILLI., .METRE. ) );
#12434=CARTESIAN_POINT ( 'NONE',  ( -11.83215956619923226, -30.00000000000000000, -4.336808689942017736E-16 ) ) ;
#12435=ORIENTED_EDGE ( 'NONE', *, *, #9778, .T. ) ;
#12449=AXIS2_PLACEMENT_3D ( 'NONE', #8183, #10157, #11218 ) ;
#12463=CARTESIAN_POINT ( 'NONE',  ( 14.00000000000000000, 30.00000000000000000, 0.000000000000000000 ) ) ;
#12475=AXIS2_PLACEMENT_3D ( 'NONE', #12125, #7417, #8250 ) ;
#12477=EDGE_LOOP ( 'NONE', ( #5547, #1976, #11048, #6158, #7390, #11459, #10608, #7842, #2158 ) ) ;
#12492=ORIENTED_EDGE ( 'NONE', *, *, #12514, .F. ) ;
#12496=AXIS2_PLACEMENT_3D ( 'NONE', #5617, #7804, #9528 ) ;
#12506=VECTOR ( 'NONE', #2174, 1000.000000000000000 ) ;
#12514=EDGE_CURVE ( 'NONE', #4835, #8365, #4786, .T. ) ;
#12524=CYLINDRICAL_SURFACE ( 'NONE', #11309, 6.000000000000000000 ) ;
#12528=ADVANCED_FACE ( 'NONE', ( #10797 ), #11783, .F. ) ;
#12535=DIRECTION ( 'NONE',  ( 0.000000000000000000, 0.000000000000000000, -1.000000000000000000 ) ) ;
#12575=CARTESIAN_POINT ( 'NONE',  ( 8.000000000000000000, 13.00000000000000178, 0.000000000000000000 ) ) ;
#12585=CARTESIAN_POINT ( 'NONE',  ( 8.000000000000000000, -13.00000000000000178, 0.000000000000000000 ) ) ;
#12600=VERTEX_POINT ( 'NONE', #4235 ) ;
#12605=VERTEX_POINT ( 'NONE', #11259 ) ;
#12618=CARTESIAN_POINT ( 'NONE',  ( 14.00000000000000000, -30.00000000000000000, -6.000000000000000000 ) ) ;
#12650=AXIS2_PLACEMENT_3D ( 'NONE', #3758, #11868, #3879 ) ;
#12659=ORIENTED_EDGE ( 'NONE', *, *, #6371, .T. ) ;
#12663=DIRECTION ( 'NONE',  ( 0.000000000000000000, 0.000000000000000000, 1.000000000000000000 ) ) ;
#12672=CIRCLE ( 'NONE', #4844, 10.00000000000000178 ) ;
#12680=CARTESIAN_POINT ( 'NONE',  ( 8.000000000000000000, 30.00000000000000000, -7.347880794884119736E-16 ) ) ;
#12709=CARTESIAN_POINT ( 'NONE',  ( 0.000000000000000000, 30.00000000000000000, 0.000000000000000000 ) ) ;
#12712=DIRECTION ( 'NONE',  ( 0.000000000000000000, 1.000000000000000000, 0.000000000000000000 ) ) ;
#12716=EDGE_CURVE ( 'NONE', #10532, #11695, #4295, .T. ) ;
#12717=LINE ( 'NONE', #2937, #3711 ) ;
#12719=EDGE_CURVE ( 'NONE', #4489, #1584, #4426, .T. ) ;
#12725=DIRECTION ( 'NONE',  ( 0.000000000000000000, 0.000000000000000000, -1.000000000000000000 ) ) ;
#12730=CARTESIAN_POINT ( 'NONE',  ( 11.17157287525379772, 30.00000000000000000, -2.828427124746177856 ) ) ;
ENDSEC;
END-ISO-10303-21;
